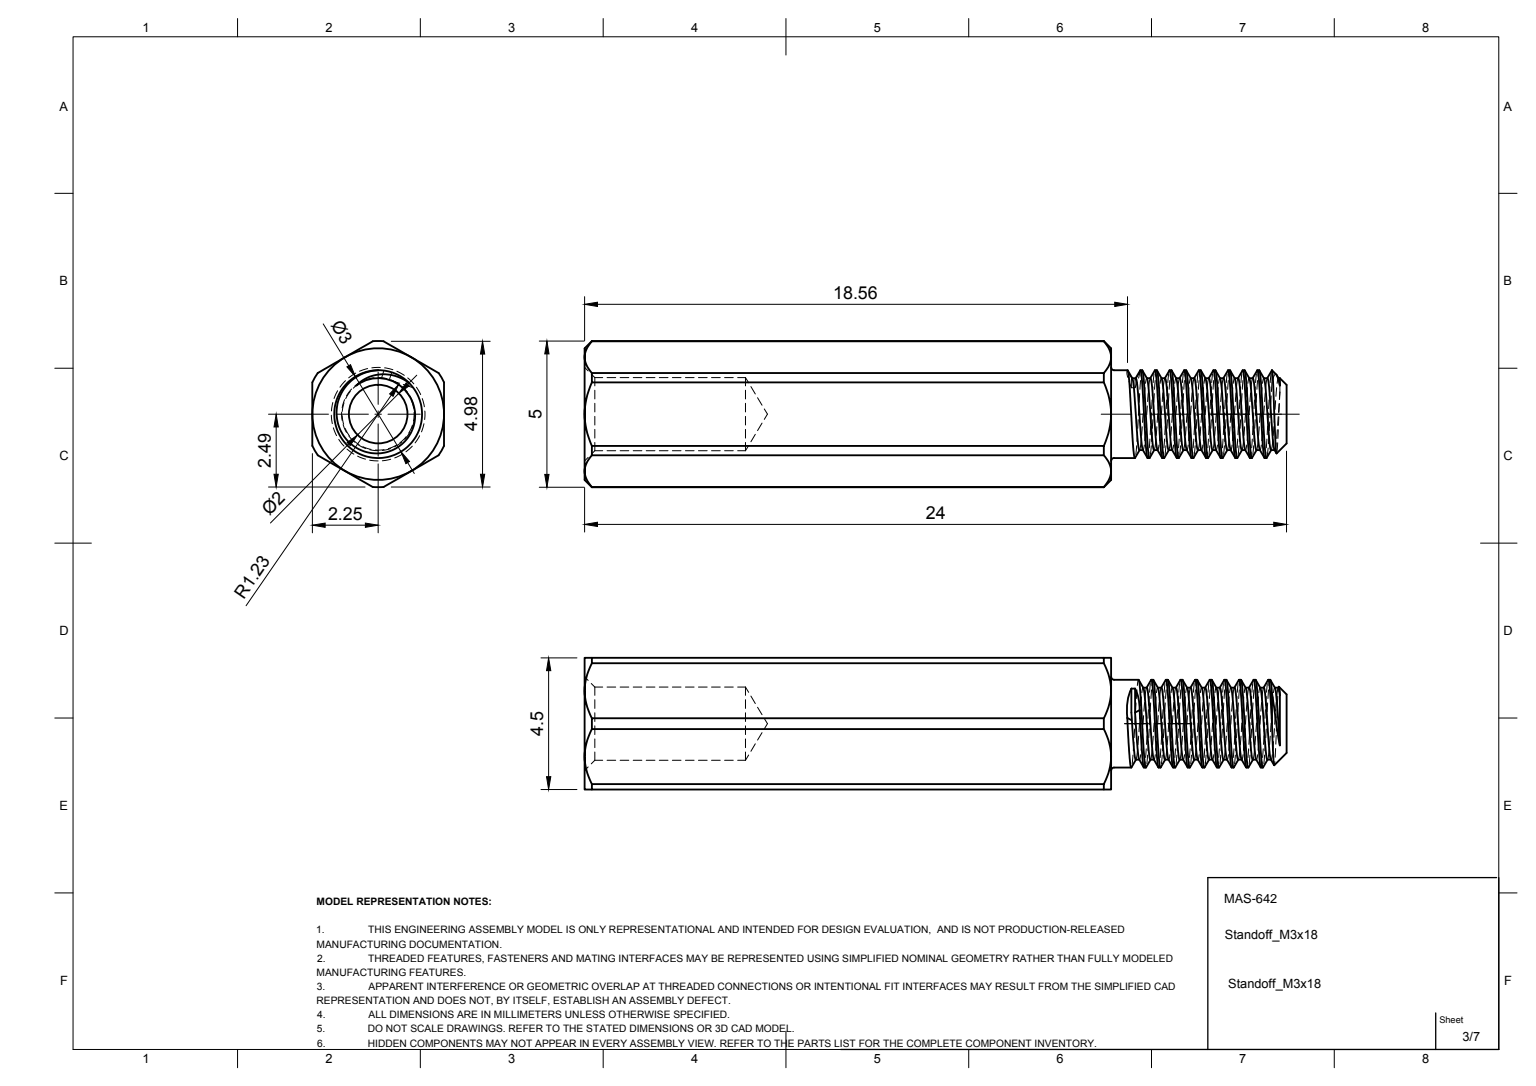
ISO-10303-21;
HEADER;
FILE_DESCRIPTION((''),'2;1');
FILE_NAME('Standoff_M3x18.step','2026-10-09T09:51:33-07:00',(''),(''),'','','');
FILE_SCHEMA (('AUTOMOTIVE_DESIGN { 1 0 10303 214 3 1 1 }'));
ENDSEC;
DATA;
#10=MECHANICAL_DESIGN_GEOMETRIC_PRESENTATION_REPRESENTATION('',(#4170),#126571);
#43=(
BOUNDED_CURVE()
B_SPLINE_CURVE(2,(#125694,#125695,#125696),.UNSPECIFIED.,.F.,.F.)
B_SPLINE_CURVE_WITH_KNOTS((3,3),(2.11928043164924,2.84165444767657),
 .UNSPECIFIED.)
CURVE()
GEOMETRIC_REPRESENTATION_ITEM()
RATIONAL_B_SPLINE_CURVE((4.94937295736919,5.22222222222224,5.22222222222224))
REPRESENTATION_ITEM('')
) ;
#44=(
BOUNDED_CURVE()
B_SPLINE_CURVE(2,(#125699,#125700,#125701),.UNSPECIFIED.,.F.,.F.)
B_SPLINE_CURVE_WITH_KNOTS((3,3),(2.84165444767658,3.56402846370389),
 .UNSPECIFIED.)
CURVE()
GEOMETRIC_REPRESENTATION_ITEM()
RATIONAL_B_SPLINE_CURVE((5.22222222222221,5.22222222222221,4.94937295736917))
REPRESENTATION_ITEM('')
) ;
#45=(
BOUNDED_CURVE()
B_SPLINE_CURVE(2,(#125705,#125706,#125707),.UNSPECIFIED.,.F.,.F.)
B_SPLINE_CURVE_WITH_KNOTS((3,3),(2.84165444767657,3.56402846370389),
 .UNSPECIFIED.)
CURVE()
GEOMETRIC_REPRESENTATION_ITEM()
RATIONAL_B_SPLINE_CURVE((5.22222222222224,5.22222222222224,4.9493729573692))
REPRESENTATION_ITEM('')
) ;
#46=(
BOUNDED_CURVE()
B_SPLINE_CURVE(2,(#125708,#125709,#125710),.UNSPECIFIED.,.F.,.F.)
B_SPLINE_CURVE_WITH_KNOTS((3,3),(2.11928043164924,2.84165444767655),
 .UNSPECIFIED.)
CURVE()
GEOMETRIC_REPRESENTATION_ITEM()
RATIONAL_B_SPLINE_CURVE((4.94937295736915,5.22222222222219,5.22222222222219))
REPRESENTATION_ITEM('')
) ;
#47=(
BOUNDED_CURVE()
B_SPLINE_CURVE(2,(#125714,#125715,#125716),.UNSPECIFIED.,.F.,.F.)
B_SPLINE_CURVE_WITH_KNOTS((3,3),(2.84165444767655,3.56402846370389),
 .UNSPECIFIED.)
CURVE()
GEOMETRIC_REPRESENTATION_ITEM()
RATIONAL_B_SPLINE_CURVE((5.22222222222219,5.22222222222219,4.94937295736914))
REPRESENTATION_ITEM('')
) ;
#48=(
BOUNDED_CURVE()
B_SPLINE_CURVE(2,(#125717,#125718,#125719),.UNSPECIFIED.,.F.,.F.)
B_SPLINE_CURVE_WITH_KNOTS((3,3),(2.11928043164923,2.84165444767657),
 .UNSPECIFIED.)
CURVE()
GEOMETRIC_REPRESENTATION_ITEM()
RATIONAL_B_SPLINE_CURVE((4.94937295736919,5.22222222222224,5.22222222222224))
REPRESENTATION_ITEM('')
) ;
#49=(
BOUNDED_CURVE()
B_SPLINE_CURVE(2,(#125723,#125724,#125725),.UNSPECIFIED.,.F.,.F.)
B_SPLINE_CURVE_WITH_KNOTS((3,3),(2.84165444767657,3.5640284637039),
 .UNSPECIFIED.)
CURVE()
GEOMETRIC_REPRESENTATION_ITEM()
RATIONAL_B_SPLINE_CURVE((5.22222222222224,5.22222222222224,4.94937295736919))
REPRESENTATION_ITEM('')
) ;
#50=(
BOUNDED_CURVE()
B_SPLINE_CURVE(2,(#125726,#125727,#125728),.UNSPECIFIED.,.F.,.F.)
B_SPLINE_CURVE_WITH_KNOTS((3,3),(2.11928043164923,2.84165444767656),
 .UNSPECIFIED.)
CURVE()
GEOMETRIC_REPRESENTATION_ITEM()
RATIONAL_B_SPLINE_CURVE((4.9493729573692,5.22222222222225,5.22222222222225))
REPRESENTATION_ITEM('')
) ;
#51=(
BOUNDED_CURVE()
B_SPLINE_CURVE(2,(#125732,#125733,#125734),.UNSPECIFIED.,.F.,.F.)
B_SPLINE_CURVE_WITH_KNOTS((3,3),(2.84165444767656,3.56402846370389),
 .UNSPECIFIED.)
CURVE()
GEOMETRIC_REPRESENTATION_ITEM()
RATIONAL_B_SPLINE_CURVE((5.22222222222225,5.22222222222225,4.94937295736921))
REPRESENTATION_ITEM('')
) ;
#52=(
BOUNDED_CURVE()
B_SPLINE_CURVE(2,(#125735,#125736,#125737),.UNSPECIFIED.,.F.,.F.)
B_SPLINE_CURVE_WITH_KNOTS((3,3),(2.11928043164924,2.84165444767656),
 .UNSPECIFIED.)
CURVE()
GEOMETRIC_REPRESENTATION_ITEM()
RATIONAL_B_SPLINE_CURVE((4.94937295736916,5.2222222222222,5.2222222222222))
REPRESENTATION_ITEM('')
) ;
#53=(
BOUNDED_CURVE()
B_SPLINE_CURVE(2,(#125740,#125741,#125742),.UNSPECIFIED.,.F.,.F.)
B_SPLINE_CURVE_WITH_KNOTS((3,3),(2.84165444767656,3.56402846370389),
 .UNSPECIFIED.)
CURVE()
GEOMETRIC_REPRESENTATION_ITEM()
RATIONAL_B_SPLINE_CURVE((5.2222222222222,5.2222222222222,4.94937295736915))
REPRESENTATION_ITEM('')
) ;
#54=(
BOUNDED_CURVE()
B_SPLINE_CURVE(2,(#125743,#125744,#125745),.UNSPECIFIED.,.F.,.F.)
B_SPLINE_CURVE_WITH_KNOTS((3,3),(2.11928043164924,2.84165444767658),
 .UNSPECIFIED.)
CURVE()
GEOMETRIC_REPRESENTATION_ITEM()
RATIONAL_B_SPLINE_CURVE((4.94937295736917,5.22222222222221,5.22222222222221))
REPRESENTATION_ITEM('')
) ;
#55=(
BOUNDED_CURVE()
B_SPLINE_CURVE(2,(#125748,#125749,#125750),.UNSPECIFIED.,.F.,.F.)
B_SPLINE_CURVE_WITH_KNOTS((3,3),(2.11928043164923,2.84165444767652),
 .UNSPECIFIED.)
CURVE()
GEOMETRIC_REPRESENTATION_ITEM()
RATIONAL_B_SPLINE_CURVE((4.94937295736913,5.22222222222216,5.22222222222217))
REPRESENTATION_ITEM('')
) ;
#56=(
BOUNDED_CURVE()
B_SPLINE_CURVE(2,(#125753,#125754,#125755),.UNSPECIFIED.,.F.,.F.)
B_SPLINE_CURVE_WITH_KNOTS((3,3),(2.84165444767653,3.56402846370387),
 .UNSPECIFIED.)
CURVE()
GEOMETRIC_REPRESENTATION_ITEM()
RATIONAL_B_SPLINE_CURVE((5.22222222222218,5.22222222222219,4.94937295736914))
REPRESENTATION_ITEM('')
) ;
#57=(
BOUNDED_CURVE()
B_SPLINE_CURVE(2,(#125759,#125760,#125761),.UNSPECIFIED.,.F.,.F.)
B_SPLINE_CURVE_WITH_KNOTS((3,3),(2.84165444767652,3.56402846370389),
 .UNSPECIFIED.)
CURVE()
GEOMETRIC_REPRESENTATION_ITEM()
RATIONAL_B_SPLINE_CURVE((5.22222222222217,5.22222222222218,4.94937295736911))
REPRESENTATION_ITEM('')
) ;
#58=(
BOUNDED_CURVE()
B_SPLINE_CURVE(2,(#125762,#125763,#125764),.UNSPECIFIED.,.F.,.F.)
B_SPLINE_CURVE_WITH_KNOTS((3,3),(2.11928043164923,2.8416544476765),
 .UNSPECIFIED.)
CURVE()
GEOMETRIC_REPRESENTATION_ITEM()
RATIONAL_B_SPLINE_CURVE((4.94937295736913,5.22222222222215,5.22222222222217))
REPRESENTATION_ITEM('')
) ;
#59=(
BOUNDED_CURVE()
B_SPLINE_CURVE(2,(#125766,#125767,#125768),.UNSPECIFIED.,.F.,.F.)
B_SPLINE_CURVE_WITH_KNOTS((3,3),(2.11928043164914,2.84165444767653),
 .UNSPECIFIED.)
CURVE()
GEOMETRIC_REPRESENTATION_ITEM()
RATIONAL_B_SPLINE_CURVE((4.94937295736908,5.22222222222217,5.22222222222218))
REPRESENTATION_ITEM('')
) ;
#60=(
BOUNDED_CURVE()
B_SPLINE_CURVE(2,(#125771,#125772,#125773),.UNSPECIFIED.,.F.,.F.)
B_SPLINE_CURVE_WITH_KNOTS((3,3),(2.84165444767655,3.5640284637039),
 .UNSPECIFIED.)
CURVE()
GEOMETRIC_REPRESENTATION_ITEM()
RATIONAL_B_SPLINE_CURVE((5.22222222222218,5.22222222222218,4.94937295736911))
REPRESENTATION_ITEM('')
) ;
#61=(
BOUNDED_CURVE()
B_SPLINE_CURVE(2,(#125775,#125776,#125777),.UNSPECIFIED.,.F.,.F.)
B_SPLINE_CURVE_WITH_KNOTS((3,3),(2.11928043164924,2.84165444767655),
 .UNSPECIFIED.)
CURVE()
GEOMETRIC_REPRESENTATION_ITEM()
RATIONAL_B_SPLINE_CURVE((4.94937295736915,5.22222222222217,5.22222222222218))
REPRESENTATION_ITEM('')
) ;
#62=(
BOUNDED_CURVE()
B_SPLINE_CURVE(2,(#125780,#125781,#125782),.UNSPECIFIED.,.F.,.F.)
B_SPLINE_CURVE_WITH_KNOTS((3,3),(2.84165444767655,3.56402846370386),
 .UNSPECIFIED.)
CURVE()
GEOMETRIC_REPRESENTATION_ITEM()
RATIONAL_B_SPLINE_CURVE((5.22222222222217,5.22222222222217,4.94937295736913))
REPRESENTATION_ITEM('')
) ;
#63=(
BOUNDED_CURVE()
B_SPLINE_CURVE(2,(#125784,#125785,#125786),.UNSPECIFIED.,.F.,.F.)
B_SPLINE_CURVE_WITH_KNOTS((3,3),(2.11928043164924,2.84165444767655),
 .UNSPECIFIED.)
CURVE()
GEOMETRIC_REPRESENTATION_ITEM()
RATIONAL_B_SPLINE_CURVE((4.94937295736914,5.22222222222217,5.22222222222217))
REPRESENTATION_ITEM('')
) ;
#64=(
BOUNDED_CURVE()
B_SPLINE_CURVE(2,(#125789,#125790,#125791),.UNSPECIFIED.,.F.,.F.)
B_SPLINE_CURVE_WITH_KNOTS((3,3),(2.84165444767657,3.56402846370392),
 .UNSPECIFIED.)
CURVE()
GEOMETRIC_REPRESENTATION_ITEM()
RATIONAL_B_SPLINE_CURVE((5.22222222222219,5.22222222222218,4.94937295736911))
REPRESENTATION_ITEM('')
) ;
#65=(
BOUNDED_CURVE()
B_SPLINE_CURVE(2,(#125793,#125794,#125795),.UNSPECIFIED.,.F.,.F.)
B_SPLINE_CURVE_WITH_KNOTS((3,3),(2.11928043164923,2.84165444767657),
 .UNSPECIFIED.)
CURVE()
GEOMETRIC_REPRESENTATION_ITEM()
RATIONAL_B_SPLINE_CURVE((4.94937295736915,5.2222222222222,5.22222222222219))
REPRESENTATION_ITEM('')
) ;
#66=(
BOUNDED_CURVE()
B_SPLINE_CURVE(2,(#125797,#125798,#125799),.UNSPECIFIED.,.F.,.F.)
B_SPLINE_CURVE_WITH_KNOTS((3,3),(2.8416544476765,3.56402846370386),
 .UNSPECIFIED.)
CURVE()
GEOMETRIC_REPRESENTATION_ITEM()
RATIONAL_B_SPLINE_CURVE((5.22222222222217,5.22222222222219,4.94937295736913))
REPRESENTATION_ITEM('')
) ;
#330=B_SPLINE_CURVE_WITH_KNOTS('',3,(#124047,#124048,#124049,#124050,#124051,
#124052,#124053,#124054,#124055,#124056,#124057,#124058,#124059,#124060,
#124061,#124062,#124063,#124064,#124065,#124066),.UNSPECIFIED.,.F.,.F.,
(4,2,2,2,2,2,2,2,2,4),(7.26097235916453,7.307487976323,7.35575594389105,
7.40257156416353,7.45158020939779,7.49931815600202,7.54681878982848,7.59584329786992,
7.64302175237609,7.68775617947263),.UNSPECIFIED.) ;
#331=B_SPLINE_CURVE_WITH_KNOTS('',3,(#124069,#124070,#124071,#124072,#124073,
#124074,#124075,#124076,#124077,#124078,#124079,#124080,#124081,#124082,
#124083,#124084,#124085,#124086,#124087,#124088),.UNSPECIFIED.,.F.,.F.,
(4,2,2,2,2,2,2,2,2,4),(0.,0.0459875521653835,0.0932819628997698,0.142429322852028,
0.189908590414643,0.237761664358612,0.28683868989661,0.333704279409584,
0.382086034209551,0.427411498485805),.UNSPECIFIED.) ;
#332=B_SPLINE_CURVE_WITH_KNOTS('',3,(#124093,#124094,#124095,#124096,#124097,
#124098,#124099,#124100,#124101,#124102,#124103,#124104,#124105,#124106,
#124107,#124108,#124109,#124110,#124111,#124112,#124113,#124114,#124115,
#124116,#124117,#124118,#124119,#124120,#124121,#124122,#124123,#124124,
#124125,#124126,#124127,#124128,#124129,#124130),.UNSPECIFIED.,.F.,.F.,
(4,2,2,2,2,2,2,2,2,2,2,2,2,2,2,2,2,2,4),(6.48467832939662,6.48870478558093,
6.53766507492409,6.58568550492772,6.63267823725172,6.68202082324882,6.72948815834683,
6.77759017644729,6.82630561099994,6.87323621682889,6.92225205593385,6.97046423370673,
7.01740641521615,7.06695661317869,7.11461532958629,7.16247212938834,7.21140015580506,
7.25849183169839,7.26097235916453),.UNSPECIFIED.) ;
#333=B_SPLINE_CURVE_WITH_KNOTS('',3,(#124131,#124132,#124133,#124134,#124135,
#124136,#124137,#124138,#124139,#124140,#124141,#124142,#124143,#124144,
#124145,#124146,#124147,#124148,#124149,#124150,#124151,#124152,#124153,
#124154,#124155,#124156,#124157,#124158,#124159,#124160,#124161,#124162,
#124163,#124164,#124165,#124166,#124167,#124168),.UNSPECIFIED.,.F.,.F.,
(4,2,2,2,2,2,2,2,2,2,2,2,2,2,2,2,2,2,4),(0.427411498485805,0.431577036060463,
0.478789185503758,0.527845315274495,0.575603226460443,0.623379302822146,
0.672502619127436,0.719463017877226,0.767773403599721,0.816880465796082,
0.864021613138868,0.912997981216,0.961170824102338,1.00888581090197,1.0584891685082,
1.10562630736056,1.1538964673421,1.20305610785317,1.20577246230604),
 .UNSPECIFIED.) ;
#334=B_SPLINE_CURVE_WITH_KNOTS('',3,(#124173,#124174,#124175,#124176,#124177,
#124178,#124179,#124180,#124181,#124182,#124183,#124184,#124185,#124186,
#124187,#124188,#124189,#124190,#124191,#124192,#124193,#124194,#124195,
#124196,#124197,#124198,#124199,#124200,#124201,#124202,#124203,#124204,
#124205,#124206,#124207,#124208),.UNSPECIFIED.,.F.,.F.,(4,2,2,2,2,2,2,2,
2,2,2,2,2,2,2,2,2,4),(5.70956420747771,5.72030972034507,5.76926273175053,
5.81700561122586,5.86434645191125,5.91338162506858,5.96056756496257,6.00942404361783,
6.05780748008125,6.10453345170252,6.15347366016584,6.20133669000566,6.24846500640859,
6.29763501900576,6.34494399136913,6.39338455386973,6.4419176261338,6.48467832939662),
 .UNSPECIFIED.) ;
#335=B_SPLINE_CURVE_WITH_KNOTS('',3,(#124209,#124210,#124211,#124212,#124213,
#124214,#124215,#124216,#124217,#124218,#124219,#124220,#124221,#124222,
#124223,#124224,#124225,#124226,#124227,#124228,#124229,#124230,#124231,
#124232,#124233,#124234,#124235,#124236,#124237,#124238,#124239,#124240,
#124241,#124242,#124243,#124244),.UNSPECIFIED.,.F.,.F.,(4,2,2,2,2,2,2,2,
2,2,2,2,2,2,2,2,2,4),(1.20577246230604,1.2500637087132,1.29884493426391,
1.34732241102889,1.39486523697925,1.44428132500633,1.49152186175626,1.53962022531109,
1.58874613172205,1.63565991568587,1.68427775017929,1.73314474249065,1.78054992698739,
1.8298155429656,1.87724047764212,1.92520328493819,1.97432941645622,1.98383043851811),
 .UNSPECIFIED.) ;
#336=B_SPLINE_CURVE_WITH_KNOTS('',3,(#124249,#124250,#124251,#124252,#124253,
#124254,#124255,#124256,#124257,#124258,#124259,#124260,#124261,#124262,
#124263,#124264,#124265,#124266,#124267,#124268,#124269,#124270,#124271,
#124272,#124273,#124274,#124275,#124276,#124277,#124278,#124279,#124280,
#124281,#124282,#124283,#124284),.UNSPECIFIED.,.F.,.F.,(4,2,2,2,2,2,2,2,
2,2,2,2,2,2,2,2,2,4),(4.93350849726113,4.95065313897434,5.0001367514161,
5.04773589353637,5.09575665066723,5.14461540943155,5.19164298059034,5.24062387411831,
5.28881904095715,5.33565288934101,5.38464956624476,5.43231220009687,5.4799267516029,
5.52886743736441,5.57596806240929,5.62529535397539,5.67356510724699,5.70956420747771),
 .UNSPECIFIED.) ;
#337=B_SPLINE_CURVE_WITH_KNOTS('',3,(#124285,#124286,#124287,#124288,#124289,
#124290,#124291,#124292,#124293,#124294,#124295,#124296,#124297,#124298,
#124299,#124300,#124301,#124302,#124303,#124304,#124305,#124306,#124307,
#124308,#124309,#124310,#124311,#124312,#124313,#124314,#124315,#124316,
#124317,#124318,#124319,#124320),.UNSPECIFIED.,.F.,.F.,(4,2,2,2,2,2,2,2,
2,2,2,2,2,2,2,2,2,4),(1.98383043851811,2.021231364205,2.0697205926988,2.11904155289011,
2.1663460448574,2.21550071170308,2.26317878691631,2.31104512794968,2.36020318829153,
2.40716845964159,2.4555671563287,2.50471172270157,2.55193271124501,2.60099435417148,
2.64904317691366,2.69683410923425,2.74652048876617,2.76242745970405),
 .UNSPECIFIED.) ;
#338=B_SPLINE_CURVE_WITH_KNOTS('',3,(#124325,#124326,#124327,#124328,#124329,
#124330,#124331,#124332,#124333,#124334,#124335,#124336,#124337,#124338,
#124339,#124340,#124341,#124342,#124343,#124344,#124345,#124346,#124347,
#124348,#124349,#124350,#124351,#124352,#124353,#124354,#124355,#124356,
#124357,#124358,#124359,#124360),.UNSPECIFIED.,.F.,.F.,(4,2,2,2,2,2,2,2,
2,2,2,2,2,2,2,2,2,4),(4.15738429453256,4.18139819511275,4.23053919796976,
4.27782394869024,4.32652355399284,4.37501975350424,4.42180928210789,4.47080187820887,
4.51878063593279,4.56588041443636,4.61517448159553,4.66259930855119,4.71091650689067,
4.7595782551651,4.80646789213435,4.8554969233847,4.90364974207811,4.93350849726113),
 .UNSPECIFIED.) ;
#339=B_SPLINE_CURVE_WITH_KNOTS('',3,(#124361,#124362,#124363,#124364,#124365,
#124366,#124367,#124368,#124369,#124370,#124371,#124372,#124373,#124374,
#124375,#124376,#124377,#124378,#124379,#124380,#124381,#124382,#124383,
#124384,#124385,#124386,#124387,#124388,#124389,#124390,#124391,#124392,
#124393,#124394,#124395,#124396),.UNSPECIFIED.,.F.,.F.,(4,2,2,2,2,2,2,2,
2,2,2,2,2,2,2,2,2,4),(2.76242745970405,2.7936241020587,2.84197026691353,
2.89114229506907,2.93820657938614,2.98705917484022,3.03536824467617,3.08297180498013,
3.13245479128841,3.17962172814637,3.22778030392872,3.27690191435427,3.32383405210944,
3.3725082345208,3.421169403163,3.46861903657913,3.51793416507266,3.54067593133588),
 .UNSPECIFIED.) ;
#340=B_SPLINE_CURVE_WITH_KNOTS('',3,(#124401,#124402,#124403,#124404,#124405,
#124406,#124407,#124408,#124409,#124410,#124411,#124412,#124413,#124414,
#124415,#124416,#124417,#124418,#124419,#124420,#124421,#124422,#124423,
#124424,#124425,#124426,#124427,#124428,#124429,#124430,#124431,#124432,
#124433,#124434,#124435,#124436),.UNSPECIFIED.,.F.,.F.,(4,2,2,2,2,2,2,2,
2,2,2,2,2,2,2,2,2,4),(3.3811260484289,3.41274900862816,3.46099351805033,
3.51004032645083,3.55700214539487,3.60575007739184,3.65387741150041,3.70137616908567,
3.75075153504194,3.79777167498976,3.84582386285438,3.89300519478398,3.94215330243098,
3.99051838064245,4.03728979359576,4.08628002368325,4.13412062890419,4.15738429453256),
 .UNSPECIFIED.) ;
#341=B_SPLINE_CURVE_WITH_KNOTS('',3,(#124437,#124438,#124439,#124440,#124441,
#124442,#124443,#124444,#124445,#124446,#124447,#124448,#124449,#124450,
#124451,#124452,#124453,#124454,#124455,#124456,#124457,#124458,#124459,
#124460,#124461,#124462,#124463,#124464,#124465,#124466,#124467,#124468,
#124469,#124470,#124471,#124472),.UNSPECIFIED.,.F.,.F.,(4,2,2,2,2,2,2,2,
2,2,2,2,2,2,2,2,2,4),(3.54067593133588,3.56524889916681,3.6132547608121,
3.66236113995851,3.70924379097633,3.75777283633892,3.80686079772826,3.85419230870826,
3.90337783950468,3.95091591719774,4.0002920934568,4.0477975955105,4.09630989433075,
4.14504988690739,4.19202367440407,4.2411602470478,4.2893880427099,4.31858521036147),
 .UNSPECIFIED.) ;
#342=B_SPLINE_CURVE_WITH_KNOTS('',3,(#124477,#124478,#124479,#124480,#124481,
#124482,#124483,#124484,#124485,#124486,#124487,#124488,#124489,#124490,
#124491,#124492,#124493,#124494,#124495,#124496,#124497,#124498,#124499,
#124500,#124501,#124502,#124503,#124504,#124505,#124506,#124507,#124508,
#124509,#124510,#124511,#124512),.UNSPECIFIED.,.F.,.F.,(4,2,2,2,2,2,2,2,
2,2,2,2,2,2,2,2,2,4),(2.60440000418254,2.64222091806599,2.69061789859203,
2.73975515555105,2.78696572159386,2.83602367520873,2.88355189021403,2.93132224967008,
2.98036249985887,3.02720769453067,3.07550834816351,3.12453618250826,3.17165958350625,
3.22062064308854,3.26850397351192,3.31619467232154,3.36577824481598,3.3811260484289),
 .UNSPECIFIED.) ;
#343=B_SPLINE_CURVE_WITH_KNOTS('',3,(#124513,#124514,#124515,#124516,#124517,
#124518,#124519,#124520,#124521,#124522,#124523,#124524,#124525,#124526,
#124527,#124528,#124529,#124530,#124531,#124532,#124533,#124534,#124535,
#124536,#124537,#124538,#124539,#124540,#124541,#124542,#124543,#124544,
#124545,#124546,#124547,#124548),.UNSPECIFIED.,.F.,.F.,(4,2,2,2,2,2,2,2,
2,2,2,2,2,2,2,2,2,4),(4.31858521036147,4.33651923363743,4.38607754453018,
4.43375037804094,4.48194507407388,4.53087577616931,4.57797363563567,4.62704987194849,
4.67531370070556,4.72225592255632,4.77134912087816,4.81907824427662,4.86684436513085,
4.91585036470624,4.96301502121423,5.01254217112715,5.06087102345235,5.09618003538743),
 .UNSPECIFIED.) ;
#344=B_SPLINE_CURVE_WITH_KNOTS('',3,(#124553,#124554,#124555,#124556,#124557,
#124558,#124559,#124560,#124561,#124562,#124563,#124564,#124565,#124566,
#124567,#124568,#124569,#124570,#124571,#124572,#124573,#124574,#124575,
#124576,#124577,#124578,#124579,#124580,#124581,#124582,#124583,#124584,
#124585,#124586,#124587,#124588),.UNSPECIFIED.,.F.,.F.,(4,2,2,2,2,2,2,2,
2,2,2,2,2,2,2,2,2,4),(1.82805130471776,1.87277646127533,1.92147530871624,
1.96979104419725,2.01725060263876,2.06658135847983,2.11369404932703,2.16170773952795,
2.2107256291696,2.25754243281317,2.30607324540708,2.35476584472025,2.40208265835429,
2.45125749765287,2.49854231366641,2.54641504154563,2.59542814286478,2.60440000418254),
 .UNSPECIFIED.) ;
#345=B_SPLINE_CURVE_WITH_KNOTS('',3,(#124589,#124590,#124591,#124592,#124593,
#124594,#124595,#124596,#124597,#124598,#124599,#124600,#124601,#124602,
#124603,#124604,#124605,#124606,#124607,#124608,#124609,#124610,#124611,
#124612,#124613,#124614,#124615,#124616,#124617,#124618,#124619,#124620,
#124621,#124622,#124623,#124624),.UNSPECIFIED.,.F.,.F.,(4,2,2,2,2,2,2,2,
2,2,2,2,2,2,2,2,2,4),(5.09618003538743,5.10770893818563,5.15675128793345,
5.20455098500115,5.25203122076791,5.3011219283047,5.34836274788015,5.39740888690433,
5.44584255805835,5.49264392480102,5.54166593188317,5.58957668485638,5.63682763234505,
5.68604400914993,5.73339928464143,5.78201352428103,5.8305888160979,5.8725887638988),
 .UNSPECIFIED.) ;
#346=B_SPLINE_CURVE_WITH_KNOTS('',3,(#124629,#124630,#124631,#124632,#124633,
#124634,#124635,#124636,#124637,#124638,#124639,#124640,#124641,#124642,
#124643,#124644,#124645,#124646,#124647,#124648,#124649,#124650,#124651,
#124652,#124653,#124654,#124655,#124656,#124657,#124658,#124659,#124660,
#124661,#124662,#124663,#124664,#124665,#124666),.UNSPECIFIED.,.F.,.F.,
(4,2,2,2,2,2,2,2,2,2,2,2,2,2,2,2,2,2,4),(1.05122908753305,1.05584848690386,
1.10298878125772,1.15197109295181,1.19959776737697,1.24730001658321,1.29632817220458,
1.34318726064785,1.39142201535752,1.44043479373918,1.48749995499297,1.536398131184,
1.58442418882633,1.63206057663025,1.68158354821496,1.72860610089148,1.77679646385941,
1.82585341919623,1.82805130471776),.UNSPECIFIED.) ;
#347=B_SPLINE_CURVE_WITH_KNOTS('',3,(#124667,#124668,#124669,#124670,#124671,
#124672,#124673,#124674,#124675,#124676,#124677,#124678,#124679,#124680,
#124681,#124682,#124683,#124684,#124685,#124686,#124687,#124688,#124689,
#124690,#124691,#124692,#124693,#124694,#124695,#124696,#124697,#124698,
#124699,#124700,#124701,#124702,#124703,#124704),.UNSPECIFIED.,.F.,.F.,
(4,2,2,2,2,2,2,2,2,2,2,2,2,2,2,2,2,2,4),(5.8725887638988,5.87743194290884,
5.92646601185683,5.97452581587684,6.02162175582692,6.07100225132472,6.11850795426233,
6.1667628942196,6.21551331591218,6.2624807124907,6.31156171305631,6.35980565105167,
6.40683027516766,6.456410610302,6.50410033527444,6.55208641404564,6.6010427526743,
6.64816284268059,6.64991209706395),.UNSPECIFIED.) ;
#348=B_SPLINE_CURVE_WITH_KNOTS('',3,(#124709,#124710,#124711,#124712,#124713,
#124714,#124715,#124716,#124717,#124718,#124719,#124720,#124721,#124722,
#124723,#124724,#124725,#124726,#124727,#124728,#124729,#124730,#124731,
#124732,#124733,#124734,#124735,#124736,#124737,#124738,#124739,#124740,
#124741,#124742,#124743,#124744),.UNSPECIFIED.,.F.,.F.,(4,2,2,2,2,2,2,2,
2,2,2,2,2,2,2,2,2,4),(0.275540243682509,0.286340819800539,0.333695388575774,
0.382913371187234,0.430062940631542,0.477971836820167,0.526948240257121,
0.573710230464671,0.622139368966846,0.670997426602599,0.718226071803216,
0.767306120243138,0.814662887431798,0.862448581964833,0.911435350682647,
0.958210116723726,1.00652260961773,1.05122908753305),.UNSPECIFIED.) ;
#349=B_SPLINE_CURVE_WITH_KNOTS('',3,(#124745,#124746,#124747,#124748,#124749,
#124750,#124751,#124752,#124753,#124754,#124755,#124756,#124757,#124758,
#124759,#124760,#124761,#124762,#124763,#124764,#124765,#124766,#124767,
#124768,#124769,#124770,#124771,#124772,#124773,#124774,#124775,#124776,
#124777,#124778,#124779,#124780),.UNSPECIFIED.,.F.,.F.,(4,2,2,2,2,2,2,2,
2,2,2,2,2,2,2,2,2,4),(6.64991209706395,6.69721143233729,6.74550549456067,
6.79238454552838,6.84144720027061,6.88920947529323,6.93681673187035,6.98586340790173,
7.03306447569406,7.08232935533034,7.13071011437757,7.17751961704142,7.22654758629657,
7.27440241377778,7.32175171314648,7.37090535322958,7.41820339493711,7.42653426035933),
 .UNSPECIFIED.) ;
#350=B_SPLINE_CURVE_WITH_KNOTS('',3,(#124786,#124787,#124788,#124789,#124790,
#124791,#124792,#124793,#124794,#124795,#124796,#124797),.UNSPECIFIED.,
 .F.,.F.,(4,2,2,2,2,4),(-0.236473027122006,-0.23458695710018,-0.176673006834002,
-0.118290109209632,-0.0588288584469845,-1.00000016489687E-6),
 .UNSPECIFIED.) ;
#351=B_SPLINE_CURVE_WITH_KNOTS('',3,(#124800,#124801,#124802,#124803,#124804,
#124805,#124806,#124807),.UNSPECIFIED.,.F.,.F.,(4,2,2,4),(-9.35462171155631,
-9.30382148989728,-9.24635104762449,-9.23530418985942),.UNSPECIFIED.) ;
#352=B_SPLINE_CURVE_WITH_KNOTS('',3,(#124812,#124813,#124814,#124815,#124816,
#124817,#124818,#124819,#124820,#124821,#124822,#124823,#124824,#124825,
#124826,#124827,#124828,#124829,#124830,#124831,#124832,#124833,#124834,
#124835,#124836,#124837,#124838,#124839,#124840,#124841,#124842,#124843,
#124844,#124845,#124846,#124847),.UNSPECIFIED.,.F.,.F.,(4,2,2,2,2,2,2,2,
2,2,2,2,2,2,2,2,2,4),(-1.1816466799126,-1.1711432489464,-1.11360549897867,
-1.05429971803153,-0.99527231100603,-0.938324784610826,-0.878701151729204,
-0.820319907036438,-0.763004488472792,-0.70301164166561,-0.645300597460547,
-0.586507743434059,-0.527276575096228,-0.470213578625258,-0.410561930645358,
-0.351974482019793,-0.294804872599786,-0.236473027122006),.UNSPECIFIED.) ;
#353=B_SPLINE_CURVE_WITH_KNOTS('',3,(#124848,#124849,#124850,#124851,#124852,
#124853,#124854,#124855,#124856,#124857,#124858,#124859,#124860,#124861,
#124862,#124863,#124864,#124865,#124866,#124867,#124868,#124869,#124870,
#124871,#124872,#124873,#124874,#124875,#124876,#124877,#124878,#124879,
#124880,#124881,#124882,#124883),.UNSPECIFIED.,.F.,.F.,(4,2,2,2,2,2,2,2,
2,2,2,2,2,2,2,2,2,4),(-9.23530418985942,-9.18662207546147,-9.1290733058091,
-9.07093314408142,-9.01135436272492,-8.95446571047789,-8.89567746304653,
-8.83575191467067,-8.77841492190154,-8.71883583043751,-8.66095591767163,
-8.60294688747092,-8.54333582365895,-8.48636391838879,-8.42770437782455,
-8.3681122074522,-8.31090295919035,-8.29087925177368),.UNSPECIFIED.) ;
#354=B_SPLINE_CURVE_WITH_KNOTS('',3,(#124888,#124889,#124890,#124891,#124892,
#124893,#124894,#124895,#124896,#124897,#124898,#124899,#124900,#124901,
#124902,#124903,#124904,#124905,#124906,#124907,#124908,#124909,#124910,
#124911,#124912,#124913,#124914,#124915,#124916,#124917,#124918,#124919,
#124920,#124921,#124922,#124923),.UNSPECIFIED.,.F.,.F.,(4,2,2,2,2,2,2,2,
2,2,2,2,2,2,2,2,2,4),(-2.12678122509193,-2.10729425304151,-2.05002580839115,
-1.99038909831469,-1.9316674048963,-1.87466417496185,-1.81501013841361,
-1.75693914324514,-1.69905824232611,-1.63941349055435,-1.58201455193184,
-1.52211994070396,-1.46326421662004,-1.40633380819462,-1.34670866487524,
-1.28850127053106,-1.2309432907053,-1.1816466799126),.UNSPECIFIED.) ;
#355=B_SPLINE_CURVE_WITH_KNOTS('',3,(#124924,#124925,#124926,#124927,#124928,
#124929,#124930,#124931,#124932,#124933,#124934,#124935,#124936,#124937,
#124938,#124939,#124940,#124941,#124942,#124943,#124944,#124945,#124946,
#124947,#124948,#124949,#124950,#124951,#124952,#124953,#124954,#124955,
#124956,#124957,#124958,#124959),.UNSPECIFIED.,.F.,.F.,(4,2,2,2,2,2,2,2,
2,2,2,2,2,2,2,2,2,4),(-8.29087925177368,-8.25146774569309,-8.1931060140114,
-8.1352172805656,-8.07502593792519,-8.01787916182783,-7.95931748219078,
-7.89969072165382,-7.84265244666734,-7.78344729198975,-7.72467517694015,
-7.66698930483589,-7.60702272505567,-7.5497294421654,-7.4913736598247,-7.43177467302502,
-7.37485108389259,-7.3459015110284),.UNSPECIFIED.) ;
#356=B_SPLINE_CURVE_WITH_KNOTS('',3,(#124964,#124965,#124966,#124967,#124968,
#124969,#124970,#124971,#124972,#124973,#124974,#124975,#124976,#124977,
#124978,#124979,#124980,#124981,#124982,#124983,#124984,#124985,#124986,
#124987,#124988,#124989,#124990,#124991,#124992,#124993,#124994,#124995,
#124996,#124997,#124998,#124999),.UNSPECIFIED.,.F.,.F.,(4,2,2,2,2,2,2,2,
2,2,2,2,2,2,2,2,2,4),(-3.07234930182782,-3.04396460692137,-2.98700170532857,
-2.92736930082992,-2.86895787619047,-2.81165872476739,-2.7516332217495,
-2.69389232736989,-2.63514802811358,-2.5758833604033,-2.51879305661577,
-2.45912888472762,-2.40050767619665,-2.34334201878956,-2.28308786627346,
-2.22514048990784,-2.16679217042194,-2.12678122509193),.UNSPECIFIED.) ;
#357=B_SPLINE_CURVE_WITH_KNOTS('',3,(#125000,#125001,#125002,#125003,#125004,
#125005,#125006,#125007,#125008,#125009,#125010,#125011,#125012,#125013,
#125014,#125015,#125016,#125017,#125018,#125019,#125020,#125021,#125022,
#125023,#125024,#125025,#125026,#125027,#125028,#125029,#125030,#125031,
#125032,#125033,#125034,#125035),.UNSPECIFIED.,.F.,.F.,(4,2,2,2,2,2,2,2,
2,2,2,2,2,2,2,2,2,4),(-7.3459015110284,-7.31584938880444,-7.25656387817681,
-7.19905098889278,-7.13927687406326,-7.08174045168678,-7.02355818700801,
-6.9639574791867,-6.90705028583207,-6.84821994204823,-6.78834540215938,
-6.73097099328063,-6.67135180647426,-6.61349209399495,-6.55544587606107,
-6.49581608898128,-6.43883548963137,-6.40128325260829),.UNSPECIFIED.) ;
#358=B_SPLINE_CURVE_WITH_KNOTS('',3,(#125040,#125041,#125042,#125043,#125044,
#125045,#125046,#125047,#125048,#125049,#125050,#125051,#125052,#125053,
#125054,#125055,#125056,#125057,#125058,#125059,#125060,#125061,#125062,
#125063,#125064,#125065,#125066,#125067,#125068,#125069,#125070,#125071,
#125072,#125073,#125074,#125075),.UNSPECIFIED.,.F.,.F.,(4,2,2,2,2,2,2,2,
2,2,2,2,2,2,2,2,2,4),(-4.01743446108088,-3.98037711695305,-3.92338026613865,
-3.86372411788194,-3.80563194583232,-3.74778671319995,-3.68811833045966,
-3.63069784236149,-3.57087032386455,-3.51198882129594,-3.45505470154523,
-3.39542422850156,-3.33719086850357,-3.27966026017497,-3.21983177136984,
-3.1622680481908,-3.10302199988204,-3.07234930182782),.UNSPECIFIED.) ;
#359=B_SPLINE_CURVE_WITH_KNOTS('',3,(#125076,#125077,#125078,#125079,#125080,
#125081,#125082,#125083,#125084,#125085,#125086,#125087,#125088,#125089,
#125090,#125091,#125092,#125093,#125094,#125095,#125096,#125097,#125098,
#125099,#125100,#125101,#125102,#125103,#125104,#125105,#125106,#125107,
#125108,#125109,#125110,#125111),.UNSPECIFIED.,.F.,.F.,(4,2,2,2,2,2,2,2,
2,2,2,2,2,2,2,2,2,4),(-6.40128325260829,-6.38013882187402,-6.32052644786668,
-6.26328232847502,-6.20380975384858,-6.14548195466263,-6.08755912059145,
-6.0273305946859,-5.97018690671393,-5.91159053837258,-5.85195029651196,
-5.79488386817085,-5.73564427374236,-5.67691979083501,-5.61920315388539,
-5.5592029693765,-5.50192507313698,-5.45600166496054),.UNSPECIFIED.) ;
#360=B_SPLINE_CURVE_WITH_KNOTS('',3,(#125116,#125117,#125118,#125119,#125120,
#125121,#125122,#125123,#125124,#125125,#125126,#125127,#125128,#125129,
#125130,#125131,#125132,#125133,#125134,#125135,#125136,#125137,#125138,
#125139,#125140,#125141,#125142,#125143,#125144,#125145,#125146,#125147,
#125148,#125149,#125150,#125151),.UNSPECIFIED.,.F.,.F.,(4,2,2,2,2,2,2,2,
2,2,2,2,2,2,2,2,2,4),(-4.96307563769018,-4.91813866664957,-4.86025738965345,
-4.80218793930441,-4.74253483237101,-4.68553219539954,-4.62681204815797,
-4.5671763186103,-4.50990933760739,-4.45041297938131,-4.3920638222817,-4.33411788796424,
-4.27386529354949,-4.21556664620729,-4.15604769936401,-4.0987601299753,
-4.03911975185839,-4.01743446108088),.UNSPECIFIED.) ;
#361=B_SPLINE_CURVE_WITH_KNOTS('',3,(#125152,#125153,#125154,#125155,#125156,
#125157,#125158,#125159,#125160,#125161,#125162,#125163,#125164,#125165,
#125166,#125167,#125168,#125169,#125170,#125171,#125172,#125173,#125174,
#125175,#125176,#125177,#125178,#125179,#125180,#125181,#125182,#125183,
#125184,#125185,#125186,#125187),.UNSPECIFIED.,.F.,.F.,(4,2,2,2,2,2,2,2,
2,2,2,2,2,2,2,2,2,4),(-5.45600166496054,-5.44353818748178,-5.38392946676581,
-5.32698965292687,-5.26795703729325,-5.20873029520478,-5.15119052229069,
-5.09138701680441,-5.03387705745448,-4.97566790823344,-4.916060903816,-4.85914913392717,
-4.80029208196713,-4.74048362398375,-4.68308675803797,-4.62463408755934,
-4.56743411515897,-4.51134022964834),.UNSPECIFIED.) ;
#362=B_SPLINE_CURVE_WITH_KNOTS('',3,(#125192,#125193,#125194,#125195,#125196,
#125197,#125198,#125199,#125200,#125201,#125202,#125203,#125204,#125205,
#125206,#125207,#125208,#125209,#125210,#125211,#125212,#125213,#125214,
#125215,#125216,#125217,#125218,#125219,#125220,#125221,#125222,#125223,
#125224,#125225,#125226,#125227),.UNSPECIFIED.,.F.,.F.,(4,2,2,2,2,2,2,2,
2,2,2,2,2,2,2,2,2,4),(-5.90797790587752,-5.85417655914304,-5.79686139893281,
-5.73848200916043,-5.67885952882914,-5.62191332079682,-5.56288777161221,
-5.50358081908249,-5.44604476955684,-5.38624654359381,-5.32868845608922,
-5.27048277087713,-5.21085866475879,-5.15392918370283,-5.0950751718008,
-5.03517915849782,-4.97778176824204,-4.96307563769018),.UNSPECIFIED.) ;
#363=B_SPLINE_CURVE_WITH_KNOTS('',3,(#125228,#125229,#125230,#125231,#125232,
#125233,#125234,#125235,#125236,#125237,#125238,#125239,#125240,#125241,
#125242,#125243,#125244,#125245,#125246,#125247,#125248,#125249,#125250,
#125251,#125252,#125253,#125254,#125255,#125256,#125257,#125258,#125259,
#125260,#125261,#125262,#125263,#125264,#125265),.UNSPECIFIED.,.F.,.F.,
(4,2,2,2,2,2,2,2,2,2,2,2,2,2,2,2,2,2,4),(-4.51134022964834,-4.50736107889285,
-4.44957955522536,-4.39103805795909,-4.33172296596087,-4.27459313534948,
-4.21494515138725,-4.15627197557177,-4.09916570838644,-4.03885333731966,
-3.98085531235153,-3.92266438621144,-3.86310737388169,-3.80578556710095,
-3.74614371498309,-3.68736332860037,-3.63038329021729,-3.57072909156752,
-3.56587391815655),.UNSPECIFIED.) ;
#364=B_SPLINE_CURVE_WITH_KNOTS('',3,(#125270,#125271,#125272,#125273,#125274,
#125275,#125276,#125277,#125278,#125279,#125280,#125281,#125282,#125283,
#125284,#125285,#125286,#125287,#125288,#125289,#125290,#125291,#125292,
#125293,#125294,#125295,#125296,#125297,#125298,#125299,#125300,#125301,
#125302,#125303,#125304,#125305,#125306,#125307),.UNSPECIFIED.,.F.,.F.,
(4,2,2,2,2,2,2,2,2,2,2,2,2,2,2,2,2,2,4),(-6.85333016178901,-6.85049761572826,
-6.79086280145887,-6.7338684673792,-6.67518502916102,-6.61556907483254,
-6.55833655807044,-6.49887713904935,-6.44049363778125,-6.38258139356379,
-6.32236555670732,-6.26519661684873,-6.20661114802352,-6.14696077866283,
-6.08989950504226,-6.03067031724312,-5.97187665370647,-5.91416744423235,
-5.90797790587752),.UNSPECIFIED.) ;
#365=B_SPLINE_CURVE_WITH_KNOTS('',3,(#125308,#125309,#125310,#125311,#125312,
#125313,#125314,#125315,#125316,#125317,#125318,#125319,#125320,#125321,
#125322,#125323,#125324,#125325,#125326,#125327,#125328,#125329,#125330,
#125331,#125332,#125333,#125334,#125335,#125336,#125337,#125338,#125339,
#125340,#125341,#125342,#125343),.UNSPECIFIED.,.F.,.F.,(4,2,2,2,2,2,2,2,
2,2,2,2,2,2,2,2,2,4),(-3.56587391815655,-3.51259862586625,-3.4548315841227,
-3.39512002261551,-3.33766052431138,-3.27797683666954,-3.21904783493571,
-3.16210893490559,-3.10247369370918,-3.04419237234846,-2.98672132744669,
-2.92683995638948,-2.86922830950958,-2.8101092431121,-2.75099595568126,
-2.69400388512544,-2.63435950322405,-2.62073726926079),.UNSPECIFIED.) ;
#366=B_SPLINE_CURVE_WITH_KNOTS('',3,(#125350,#125351,#125352,#125353,#125354,
#125355,#125356,#125357,#125358,#125359,#125360,#125361,#125362,#125363,
#125364,#125365,#125366,#125367,#125368,#125369,#125370,#125371,#125372,
#125373,#125374,#125375,#125376,#125377),.UNSPECIFIED.,.F.,.F.,(4,2,2,2,
2,2,2,2,2,2,2,2,2,4),(-0.729144904376339,-0.701294765627904,-0.644290240572763,
-0.584622721852303,-0.526155163852952,-0.468846061685899,-0.408761237620433,
-0.350964868034901,-0.292242330555774,-0.23291790866579,-0.175774000270549,
-0.116070886581869,-0.0573899304566333,0.),.UNSPECIFIED.) ;
#367=B_SPLINE_CURVE_WITH_KNOTS('',3,(#125385,#125386,#125387,#125388,#125389,
#125390,#125391,#125392,#125393,#125394,#125395,#125396,#125397,#125398,
#125399,#125400,#125401,#125402,#125403,#125404,#125405,#125406,#125407,
#125408,#125409,#125410,#125411,#125412,#125413,#125414),.UNSPECIFIED.,
 .F.,.F.,(4,2,2,2,2,2,2,2,2,2,2,2,2,2,4),(-8.55374923263164,-8.52045997548488,
-8.48812186400397,-8.43025873621608,-8.37009569721686,-8.31293715613035,
-8.25440154797182,-8.19477991623858,-8.1377605421172,-8.07858114325935,
-8.01975349658949,-7.96208993347597,-7.90214811438955,-7.84483111171218,
-7.79788942893258),.UNSPECIFIED.) ;
#368=B_SPLINE_CURVE_WITH_KNOTS('',3,(#125417,#125418,#125419,#125420,#125421,
#125422,#125423,#125424,#125425,#125426,#125427,#125428,#125429,#125430,
#125431,#125432,#125433,#125434,#125435,#125436,#125437,#125438,#125439,
#125440,#125441,#125442,#125443,#125444,#125445,#125446,#125447,#125448,
#125449,#125450,#125451,#125452),.UNSPECIFIED.,.F.,.F.,(4,2,2,2,2,2,2,2,
2,2,2,2,2,2,2,2,2,4),(-1.67472695159199,-1.63814253054756,-1.58112626326033,
-1.52144174075491,-1.46330248400391,-1.40546717323888,-1.34574854931093,
-1.28828093672951,-1.228494242623,-1.1695607477854,-1.11259684987605,-1.05293475628546,
-0.994649499089507,-0.937120115226852,-0.877236543088398,-0.819621249528116,
-0.760408371557094,-0.729144904376339),.UNSPECIFIED.) ;
#369=B_SPLINE_CURVE_WITH_KNOTS('',3,(#125454,#125455,#125456,#125457,#125458,
#125459,#125460,#125461,#125462,#125463,#125464,#125465,#125466,#125467,
#125468,#125469,#125470,#125471,#125472,#125473,#125474,#125475,#125476,
#125477,#125478,#125479,#125480,#125481,#125482,#125483,#125484,#125485,
#125486,#125487,#125488,#125489),.UNSPECIFIED.,.F.,.F.,(4,2,2,2,2,2,2,2,
2,2,2,2,2,2,2,2,2,4),(-7.79788942893258,-7.7864978331053,-7.72690027532479,
-7.66998381914493,-7.61100430828218,-7.55165262671408,-7.49415813115462,
-7.434404527004,-7.37683370109388,-7.31866970220167,-7.25906709251872,-7.20215576863061,
-7.14334343176941,-7.08339598828515,-7.02603560425023,-6.96643217276498,
-6.9085302919768,-6.85333016178901),.UNSPECIFIED.) ;
#370=B_SPLINE_CURVE_WITH_KNOTS('',3,(#125490,#125491,#125492,#125493,#125494,
#125495,#125496,#125497,#125498,#125499,#125500,#125501,#125502,#125503,
#125504,#125505,#125506,#125507,#125508,#125509,#125510,#125511,#125512,
#125513,#125514,#125515,#125516,#125517,#125518,#125519,#125520,#125521,
#125522,#125523,#125524,#125525),.UNSPECIFIED.,.F.,.F.,(4,2,2,2,2,2,2,2,
2,2,2,2,2,2,2,2,2,4),(-2.62073726926079,-2.57589168419096,-2.51862873581428,
-2.45854193473685,-2.40074535328825,-2.34210369906827,-2.28277616139501,
-2.22563231373495,-2.16594829107943,-2.10726356038932,-2.05010847618233,
-1.98978591242265,-1.93177619281583,-1.87350153298898,-1.81393494970357,
-1.75660268268265,-1.69693230395467,-1.67472695159199),.UNSPECIFIED.) ;
#371=B_SPLINE_CURVE_WITH_KNOTS('',3,(#125528,#125529,#125530,#125531,#125532,
#125533,#125534,#125535,#125536,#125537,#125538,#125539,#125540,#125541,
#125542,#125543,#125544,#125545,#125546,#125547,#125548,#125549),
 .UNSPECIFIED.,.F.,.F.,(4,2,2,2,2,2,2,2,2,2,4),(7.42653426035933,7.46701042314504,
7.51551605666961,7.56232997551886,7.61135461607121,7.65934114232017,7.70649931554284,
7.75579949517463,7.80323150261535,7.848007974901,7.89462988945302),
 .UNSPECIFIED.) ;
#372=B_SPLINE_CURVE_WITH_KNOTS('',3,(#125552,#125553,#125554,#125555,#125556,
#125557,#125558,#125559,#125560,#125561,#125562,#125563,#125564,#125565),
 .UNSPECIFIED.,.F.,.F.,(4,2,2,2,2,2,4),(9.99999999993084E-7,0.0454152741647829,
0.0934842511977,0.142483198960695,0.189312581462748,0.237893912869686,0.275540243682509),
 .UNSPECIFIED.) ;
#373=B_SPLINE_CURVE_WITH_KNOTS('',3,(#125585,#125586,#125587,#125588,#125589,
#125590,#125591,#125592,#125593,#125594,#125595,#125596,#125597,#125598,
#125599,#125600,#125601,#125602,#125603,#125604,#125605,#125606,#125607,
#125608,#125609,#125610,#125611,#125612,#125613,#125614),.UNSPECIFIED.,
 .F.,.F.,(4,2,2,2,2,2,2,2,2,2,2,2,2,2,4),(0.102793946330879,0.14065908540827,
0.207546049472987,0.277181081921595,0.341925843104979,0.425232051113792,
0.529553206832786,0.635138456761143,0.687061075445346,0.791098170318975,
0.901479157744014,1.02330053588931,1.15825935025609,1.22953088710868,1.29476085683451),
 .UNSPECIFIED.) ;
#374=B_SPLINE_CURVE_WITH_KNOTS('',3,(#125618,#125619,#125620,#125621,#125622,
#125623,#125624,#125625),.UNSPECIFIED.,.F.,.F.,(4,2,2,4),(0.,0.0368526993038302,
0.0772866279385214,0.102793946330879),.UNSPECIFIED.) ;
#375=B_SPLINE_CURVE_WITH_KNOTS('',3,(#125626,#125627,#125628,#125629,#125630,
#125631,#125632,#125633,#125634,#125635,#125636,#125637),.UNSPECIFIED.,
 .F.,.F.,(4,2,2,2,2,4),(-0.166237454912908,-0.14614759649084,-0.124790609402371,
-0.083627563805611,-0.0424146450456111,0.),.UNSPECIFIED.) ;
#376=B_SPLINE_CURVE_WITH_KNOTS('',3,(#126352,#126353,#126354,#126355,#126356,
#126357,#126358,#126359,#126360,#126361),.UNSPECIFIED.,.F.,.F.,(4,3,3,4),
(0.,8.73464104464917E-5,0.000174692824679549,0.000283410104056903),
 .UNSPECIFIED.) ;
#467=(
BOUNDED_SURFACE()
B_SPLINE_SURFACE(1,2,((#125809,#125810,#125811,#125812,#125813,#125814,
#125815,#125816,#125817,#125818,#125819,#125820,#125821,#125822,#125823,
#125824,#125825,#125826,#125827,#125828,#125829,#125830,#125831,#125832,
#125833,#125834,#125835,#125836,#125837,#125838,#125839,#125840,#125841,
#125842,#125843,#125844,#125845,#125846,#125847,#125848,#125849,#125850,
#125851,#125852,#125853,#125854,#125855,#125856,#125857,#125858,#125859,
#125860,#125861,#125862,#125863,#125864,#125865,#125866,#125867,#125868,
#125869,#125870,#125871,#125872,#125873,#125874,#125875,#125876,#125877,
#125878,#125879,#125880,#125881,#125882,#125883,#125884,#125885,#125886,
#125887,#125888,#125889,#125890,#125891,#125892,#125893,#125894,#125895,
#125896,#125897,#125898,#125899,#125900,#125901,#125902,#125903,#125904,
#125905,#125906,#125907,#125908,#125909,#125910,#125911,#125912,#125913,
#125914,#125915,#125916,#125917,#125918,#125919,#125920,#125921,#125922,
#125923,#125924,#125925,#125926,#125927,#125928,#125929,#125930,#125931,
#125932,#125933,#125934,#125935,#125936,#125937,#125938,#125939,#125940,
#125941,#125942,#125943),(#125944,#125945,#125946,#125947,#125948,#125949,
#125950,#125951,#125952,#125953,#125954,#125955,#125956,#125957,#125958,
#125959,#125960,#125961,#125962,#125963,#125964,#125965,#125966,#125967,
#125968,#125969,#125970,#125971,#125972,#125973,#125974,#125975,#125976,
#125977,#125978,#125979,#125980,#125981,#125982,#125983,#125984,#125985,
#125986,#125987,#125988,#125989,#125990,#125991,#125992,#125993,#125994,
#125995,#125996,#125997,#125998,#125999,#126000,#126001,#126002,#126003,
#126004,#126005,#126006,#126007,#126008,#126009,#126010,#126011,#126012,
#126013,#126014,#126015,#126016,#126017,#126018,#126019,#126020,#126021,
#126022,#126023,#126024,#126025,#126026,#126027,#126028,#126029,#126030,
#126031,#126032,#126033,#126034,#126035,#126036,#126037,#126038,#126039,
#126040,#126041,#126042,#126043,#126044,#126045,#126046,#126047,#126048,
#126049,#126050,#126051,#126052,#126053,#126054,#126055,#126056,#126057,
#126058,#126059,#126060,#126061,#126062,#126063,#126064,#126065,#126066,
#126067,#126068,#126069,#126070,#126071,#126072,#126073,#126074,#126075,
#126076,#126077,#126078)),.UNSPECIFIED.,.F.,.F.,.F.)
B_SPLINE_SURFACE_WITH_KNOTS((2,2),(3,2,2,2,2,2,2,2,2,2,2,2,2,2,2,2,2,2,
2,2,2,2,2,2,2,2,2,2,2,2,2,2,2,2,2,2,2,2,2,2,2,2,2,2,2,2,2,2,2,2,2,2,2,2,
2,2,2,2,2,2,2,2,2,2,2,2,2,3),(0.,1.00006111776867),(0.,0.0138888888888889,
0.0277777777777778,0.0416666666666667,0.0555555555555556,0.0694444444444444,
0.0833333333333333,0.0972222222222222,0.111111111111111,0.125,0.138888888888889,
0.152777777777778,0.166666666666667,0.180555555555556,0.194444444444444,
0.208333333333333,0.222222222222222,0.236111111111111,0.25,0.263888888888889,
0.277777777777778,0.291666666666667,0.305555555555556,0.319444444444444,
0.333333333333333,0.347222222222222,0.361111111111111,0.375,0.388888888888889,
0.402777777777778,0.416666666666667,0.430555555555556,0.444444444444444,
0.458333333333333,0.472222222222222,0.486111111111111,0.5,0.513888888888889,
0.527777777777778,0.541666666666667,0.555555555555556,0.569444444444444,
0.583333333333333,0.597222222222222,0.611111111111111,0.625,0.638888888888889,
0.652777777777778,0.666666666666667,0.680555555555556,0.694444444444444,
0.708333333333333,0.722222222222222,0.736111111111111,0.75,0.763888888888889,
0.777777777777778,0.791666666666667,0.805555555555556,0.819444444444444,
0.833333333333333,0.847222222222222,0.861111111111111,0.875,0.888888888888889,
0.902777777777778,0.916666666666667,0.920887586444199),.UNSPECIFIED.)
GEOMETRIC_REPRESENTATION_ITEM()
RATIONAL_B_SPLINE_SURFACE(((1.,0.866025403784439,1.,0.866025403784439,1.,
0.866025403784439,1.,0.866025403784439,1.,0.866025403784439,1.,0.866025403784439,
1.,0.866025403784439,1.,0.866025403784439,1.,0.866025403784439,1.,0.866025403784439,
1.,0.866025403784439,1.,0.866025403784439,1.,0.866025403784439,1.,0.866025403784439,
1.,0.866025403784439,1.,0.866025403784439,1.,0.866025403784439,1.,0.866025403784439,
1.,0.866025403784439,1.,0.866025403784439,1.,0.866025403784439,1.,0.866025403784439,
1.,0.866025403784439,1.,0.866025403784439,1.,0.866025403784439,1.,0.866025403784439,
1.,0.866025403784439,1.,0.866025403784439,1.,0.866025403784439,1.,0.866025403784439,
1.,0.866025403784439,1.,0.866025403784439,1.,0.866025403784439,1.,0.866025403784439,
1.,0.866025403784439,1.,0.866025403784439,1.,0.866025403784439,1.,0.866025403784439,
1.,0.866025403784439,1.,0.866025403784439,1.,0.866025403784439,1.,0.866025403784439,
1.,0.866025403784439,1.,0.866025403784439,1.,0.866025403784439,1.,0.866025403784439,
1.,0.866025403784439,1.,0.866025403784439,1.,0.866025403784439,1.,0.866025403784439,
1.,0.866025403784439,1.,0.866025403784439,1.,0.866025403784439,1.,0.866025403784439,
1.,0.866025403784439,1.,0.866025403784439,1.,0.866025403784439,1.,0.866025403784439,
1.,0.866025403784439,1.,0.866025403784439,1.,0.866025403784439,1.,0.866025403784439,
1.,0.866025403784439,1.,0.866025403784439,1.,0.866025403784439,1.,0.866025403784439,
1.,0.959284286354576,0.943316090290602),(1.,0.866025403784439,1.,0.866025403784439,
1.,0.866025403784439,1.,0.866025403784439,1.,0.866025403784439,1.,0.866025403784439,
1.,0.866025403784439,1.,0.866025403784439,1.,0.866025403784439,1.,0.866025403784439,
1.,0.866025403784439,1.,0.866025403784439,1.,0.866025403784439,1.,0.866025403784439,
1.,0.866025403784439,1.,0.866025403784439,1.,0.866025403784439,1.,0.866025403784439,
1.,0.866025403784439,1.,0.866025403784439,1.,0.866025403784439,1.,0.866025403784439,
1.,0.866025403784439,1.,0.866025403784439,1.,0.866025403784439,1.,0.866025403784439,
1.,0.866025403784439,1.,0.866025403784439,1.,0.866025403784439,1.,0.866025403784439,
1.,0.866025403784439,1.,0.866025403784439,1.,0.866025403784439,1.,0.866025403784439,
1.,0.866025403784439,1.,0.866025403784439,1.,0.866025403784439,1.,0.866025403784439,
1.,0.866025403784439,1.,0.866025403784439,1.,0.866025403784439,1.,0.866025403784439,
1.,0.866025403784439,1.,0.866025403784439,1.,0.866025403784439,1.,0.866025403784439,
1.,0.866025403784439,1.,0.866025403784439,1.,0.866025403784439,1.,0.866025403784439,
1.,0.866025403784439,1.,0.866025403784439,1.,0.866025403784439,1.,0.866025403784439,
1.,0.866025403784439,1.,0.866025403784439,1.,0.866025403784439,1.,0.866025403784439,
1.,0.866025403784439,1.,0.866025403784439,1.,0.866025403784439,1.,0.866025403784439,
1.,0.866025403784439,1.,0.866025403784439,1.,0.866025403784439,1.,0.866025403784439,
1.,0.959284286354576,0.943316090290602)))
REPRESENTATION_ITEM('')
SURFACE()
) ;
#468=(
BOUNDED_SURFACE()
B_SPLINE_SURFACE(1,2,((#126080,#126081,#126082,#126083,#126084,#126085,
#126086,#126087,#126088,#126089,#126090,#126091,#126092,#126093,#126094,
#126095,#126096,#126097,#126098,#126099,#126100,#126101,#126102,#126103,
#126104,#126105,#126106,#126107,#126108,#126109,#126110,#126111,#126112,
#126113,#126114,#126115,#126116,#126117,#126118,#126119,#126120,#126121,
#126122,#126123,#126124,#126125,#126126,#126127,#126128,#126129,#126130,
#126131,#126132,#126133,#126134,#126135,#126136,#126137,#126138,#126139,
#126140,#126141,#126142,#126143,#126144,#126145,#126146,#126147,#126148,
#126149,#126150,#126151,#126152,#126153,#126154,#126155,#126156,#126157,
#126158,#126159,#126160,#126161,#126162,#126163,#126164,#126165,#126166,
#126167,#126168,#126169,#126170,#126171,#126172,#126173,#126174,#126175,
#126176,#126177,#126178,#126179,#126180,#126181,#126182,#126183,#126184,
#126185,#126186,#126187,#126188,#126189,#126190,#126191,#126192,#126193,
#126194,#126195,#126196,#126197,#126198,#126199,#126200,#126201,#126202,
#126203,#126204,#126205,#126206,#126207,#126208,#126209,#126210,#126211,
#126212,#126213,#126214),(#126215,#126216,#126217,#126218,#126219,#126220,
#126221,#126222,#126223,#126224,#126225,#126226,#126227,#126228,#126229,
#126230,#126231,#126232,#126233,#126234,#126235,#126236,#126237,#126238,
#126239,#126240,#126241,#126242,#126243,#126244,#126245,#126246,#126247,
#126248,#126249,#126250,#126251,#126252,#126253,#126254,#126255,#126256,
#126257,#126258,#126259,#126260,#126261,#126262,#126263,#126264,#126265,
#126266,#126267,#126268,#126269,#126270,#126271,#126272,#126273,#126274,
#126275,#126276,#126277,#126278,#126279,#126280,#126281,#126282,#126283,
#126284,#126285,#126286,#126287,#126288,#126289,#126290,#126291,#126292,
#126293,#126294,#126295,#126296,#126297,#126298,#126299,#126300,#126301,
#126302,#126303,#126304,#126305,#126306,#126307,#126308,#126309,#126310,
#126311,#126312,#126313,#126314,#126315,#126316,#126317,#126318,#126319,
#126320,#126321,#126322,#126323,#126324,#126325,#126326,#126327,#126328,
#126329,#126330,#126331,#126332,#126333,#126334,#126335,#126336,#126337,
#126338,#126339,#126340,#126341,#126342,#126343,#126344,#126345,#126346,
#126347,#126348,#126349)),.UNSPECIFIED.,.F.,.F.,.F.)
B_SPLINE_SURFACE_WITH_KNOTS((2,2),(3,2,2,2,2,2,2,2,2,2,2,2,2,2,2,2,2,2,
2,2,2,2,2,2,2,2,2,2,2,2,2,2,2,2,2,2,2,2,2,2,2,2,2,2,2,2,2,2,2,2,2,2,2,2,
2,2,2,2,2,2,2,2,2,2,2,2,2,3),(0.,1.),(0.,0.0138888888888889,0.0277777777777778,
0.0416666666666667,0.0555555555555556,0.0694444444444444,0.0833333333333333,
0.0972222222222222,0.111111111111111,0.125,0.138888888888889,0.152777777777778,
0.166666666666667,0.180555555555556,0.194444444444444,0.208333333333333,
0.222222222222222,0.236111111111111,0.25,0.263888888888889,0.277777777777778,
0.291666666666667,0.305555555555556,0.319444444444444,0.333333333333333,
0.347222222222222,0.361111111111111,0.375,0.388888888888889,0.402777777777778,
0.416666666666667,0.430555555555556,0.444444444444444,0.458333333333333,
0.472222222222222,0.486111111111111,0.5,0.513888888888889,0.527777777777778,
0.541666666666667,0.555555555555556,0.569444444444444,0.583333333333333,
0.597222222222222,0.611111111111111,0.625,0.638888888888889,0.652777777777778,
0.666666666666667,0.680555555555556,0.694444444444444,0.708333333333333,
0.722222222222222,0.736111111111111,0.75,0.763888888888889,0.777777777777778,
0.791666666666667,0.805555555555556,0.819444444444444,0.833333333333333,
0.847222222222222,0.861111111111111,0.875,0.888888888888889,0.902777777777778,
0.916666666666667,0.920887434615967),.UNSPECIFIED.)
GEOMETRIC_REPRESENTATION_ITEM()
RATIONAL_B_SPLINE_SURFACE(((1.,0.866025403784439,1.,0.866025403784439,1.,
0.866025403784439,1.,0.866025403784439,1.,0.866025403784439,1.,0.866025403784439,
1.,0.866025403784439,1.,0.866025403784439,1.,0.866025403784439,1.,0.866025403784439,
1.,0.866025403784439,1.,0.866025403784439,1.,0.866025403784439,1.,0.866025403784439,
1.,0.866025403784439,1.,0.866025403784439,1.,0.866025403784439,1.,0.866025403784439,
1.,0.866025403784439,1.,0.866025403784439,1.,0.866025403784439,1.,0.866025403784439,
1.,0.866025403784439,1.,0.866025403784439,1.,0.866025403784439,1.,0.866025403784439,
1.,0.866025403784439,1.,0.866025403784439,1.,0.866025403784439,1.,0.866025403784439,
1.,0.866025403784439,1.,0.866025403784439,1.,0.866025403784439,1.,0.866025403784439,
1.,0.866025403784439,1.,0.866025403784439,1.,0.866025403784439,1.,0.866025403784439,
1.,0.866025403784439,1.,0.866025403784439,1.,0.866025403784439,1.,0.866025403784439,
1.,0.866025403784439,1.,0.866025403784439,1.,0.866025403784439,1.,0.866025403784439,
1.,0.866025403784439,1.,0.866025403784439,1.,0.866025403784439,1.,0.866025403784439,
1.,0.866025403784439,1.,0.866025403784439,1.,0.866025403784439,1.,0.866025403784439,
1.,0.866025403784439,1.,0.866025403784439,1.,0.866025403784439,1.,0.866025403784439,
1.,0.866025403784439,1.,0.866025403784439,1.,0.866025403784439,1.,0.866025403784439,
1.,0.866025403784439,1.,0.866025403784439,1.,0.866025403784439,1.,0.866025403784439,
1.,0.959285750915652,0.943317239087869),(1.,0.866025403784439,1.,0.866025403784439,
1.,0.866025403784439,1.,0.866025403784439,1.,0.866025403784439,1.,0.866025403784439,
1.,0.866025403784439,1.,0.866025403784439,1.,0.866025403784439,1.,0.866025403784439,
1.,0.866025403784439,1.,0.866025403784439,1.,0.866025403784439,1.,0.866025403784439,
1.,0.866025403784439,1.,0.866025403784439,1.,0.866025403784439,1.,0.866025403784439,
1.,0.866025403784439,1.,0.866025403784439,1.,0.866025403784439,1.,0.866025403784439,
1.,0.866025403784439,1.,0.866025403784439,1.,0.866025403784439,1.,0.866025403784439,
1.,0.866025403784439,1.,0.866025403784439,1.,0.866025403784439,1.,0.866025403784439,
1.,0.866025403784439,1.,0.866025403784439,1.,0.866025403784439,1.,0.866025403784439,
1.,0.866025403784439,1.,0.866025403784439,1.,0.866025403784439,1.,0.866025403784439,
1.,0.866025403784439,1.,0.866025403784439,1.,0.866025403784439,1.,0.866025403784439,
1.,0.866025403784439,1.,0.866025403784439,1.,0.866025403784439,1.,0.866025403784439,
1.,0.866025403784439,1.,0.866025403784439,1.,0.866025403784439,1.,0.866025403784439,
1.,0.866025403784439,1.,0.866025403784439,1.,0.866025403784439,1.,0.866025403784439,
1.,0.866025403784439,1.,0.866025403784439,1.,0.866025403784439,1.,0.866025403784439,
1.,0.866025403784439,1.,0.866025403784439,1.,0.866025403784439,1.,0.866025403784439,
1.,0.866025403784439,1.,0.866025403784439,1.,0.866025403784439,1.,0.866025403784439,
1.,0.959285750915652,0.943317239087869)))
REPRESENTATION_ITEM('')
SURFACE()
) ;
#473=SHAPE_REPRESENTATION_RELATIONSHIP('SRR','None',#126603,#479) ;
#479=ADVANCED_BREP_SHAPE_REPRESENTATION('',(#4180),#126569) ;
#4170=STYLED_ITEM('',(#126644),#4180) ;
#4180=MANIFOLD_SOLID_BREP('Body1',#67694) ;
#4983=ELLIPSE('',#76691,1.73204548364451,1.5) ;
#4984=ELLIPSE('',#76692,1.73205681329418,1.5) ;
#5061=FACE_BOUND('',#24666,.T.) ;
#5062=FACE_BOUND('',#24668,.T.) ;
#5913=PLANE('',#76749) ;
#5914=PLANE('',#76750) ;
#5915=PLANE('',#76751) ;
#5916=PLANE('',#76752) ;
#5917=PLANE('',#76753) ;
#5918=PLANE('',#76754) ;
#5919=PLANE('',#76755) ;
#5920=PLANE('',#76756) ;
#5921=PLANE('',#76757) ;
#5922=PLANE('',#76759) ;
#5923=PLANE('',#76760) ;
#5924=PLANE('',#76761) ;
#7866=CYLINDRICAL_SURFACE('',#76670,1.2293670625) ;
#7867=CYLINDRICAL_SURFACE('',#76671,1.2293670625) ;
#7868=CYLINDRICAL_SURFACE('',#76672,1.2293670625) ;
#7869=CYLINDRICAL_SURFACE('',#76673,1.2293670625) ;
#7870=CYLINDRICAL_SURFACE('',#76674,1.2293670625) ;
#7871=CYLINDRICAL_SURFACE('',#76675,1.2293670625) ;
#7872=CYLINDRICAL_SURFACE('',#76676,1.2293670625) ;
#7873=CYLINDRICAL_SURFACE('',#76677,1.2293670625) ;
#7874=CYLINDRICAL_SURFACE('',#76678,1.2293670625) ;
#7875=CYLINDRICAL_SURFACE('',#76679,1.2293670625) ;
#7876=CYLINDRICAL_SURFACE('',#76680,1.5) ;
#7877=CYLINDRICAL_SURFACE('',#76682,1.5) ;
#7878=CYLINDRICAL_SURFACE('',#76683,1.5) ;
#7879=CYLINDRICAL_SURFACE('',#76684,1.5) ;
#7880=CYLINDRICAL_SURFACE('',#76685,1.5) ;
#7881=CYLINDRICAL_SURFACE('',#76686,1.5) ;
#7882=CYLINDRICAL_SURFACE('',#76687,1.5) ;
#7883=CYLINDRICAL_SURFACE('',#76688,1.5) ;
#7884=CYLINDRICAL_SURFACE('',#76689,1.5) ;
#7885=CYLINDRICAL_SURFACE('',#76693,1.5) ;
#7886=CYLINDRICAL_SURFACE('',#76694,1.2293670625) ;
#7887=CYLINDRICAL_SURFACE('',#76699,1.25) ;
#7888=CYLINDRICAL_SURFACE('',#76707,2.49807621135332) ;
#7889=CYLINDRICAL_SURFACE('',#76710,2.49807621135332) ;
#7890=CYLINDRICAL_SURFACE('',#76713,2.49807621135332) ;
#7891=CYLINDRICAL_SURFACE('',#76716,2.49807621135332) ;
#7892=CYLINDRICAL_SURFACE('',#76719,2.49807621135332) ;
#7893=CYLINDRICAL_SURFACE('',#76722,2.49807621135332) ;
#11944=LINE('',#124045,#16060) ;
#11945=LINE('',#124068,#16061) ;
#11946=LINE('',#124092,#16062) ;
#11947=LINE('',#124172,#16063) ;
#11948=LINE('',#124248,#16064) ;
#11949=LINE('',#124324,#16065) ;
#11950=LINE('',#124400,#16066) ;
#11951=LINE('',#124476,#16067) ;
#11952=LINE('',#124552,#16068) ;
#11953=LINE('',#124628,#16069) ;
#11954=LINE('',#124708,#16070) ;
#11955=LINE('',#124784,#16071) ;
#11956=LINE('',#124811,#16072) ;
#11957=LINE('',#124887,#16073) ;
#11958=LINE('',#124963,#16074) ;
#11959=LINE('',#125039,#16075) ;
#11960=LINE('',#125115,#16076) ;
#11961=LINE('',#125191,#16077) ;
#11962=LINE('',#125269,#16078) ;
#11963=LINE('',#125348,#16079) ;
#11964=LINE('',#125381,#16080) ;
#11965=LINE('',#125416,#16081) ;
#11966=LINE('',#125570,#16082) ;
#11967=LINE('',#125575,#16083) ;
#11968=LINE('',#125578,#16084) ;
#11969=LINE('',#125616,#16085) ;
#11970=LINE('',#125641,#16086) ;
#11971=LINE('',#125645,#16087) ;
#11972=LINE('',#125650,#16088) ;
#11973=LINE('',#125654,#16089) ;
#11974=LINE('',#125659,#16090) ;
#11975=LINE('',#125663,#16091) ;
#11976=LINE('',#125668,#16092) ;
#11977=LINE('',#125672,#16093) ;
#11978=LINE('',#125677,#16094) ;
#11979=LINE('',#125681,#16095) ;
#11980=LINE('',#125686,#16096) ;
#11981=LINE('',#125690,#16097) ;
#11982=LINE('',#126079,#16098) ;
#11983=LINE('',#126363,#16099) ;
#11984=LINE('',#126365,#16100) ;
#16060=VECTOR('',#98716,1.2293670625) ;
#16061=VECTOR('',#98717,10.) ;
#16062=VECTOR('',#98720,1.2293670625) ;
#16063=VECTOR('',#98723,1.2293670625) ;
#16064=VECTOR('',#98726,1.2293670625) ;
#16065=VECTOR('',#98729,1.2293670625) ;
#16066=VECTOR('',#98732,1.2293670625) ;
#16067=VECTOR('',#98735,1.2293670625) ;
#16068=VECTOR('',#98738,1.2293670625) ;
#16069=VECTOR('',#98741,1.2293670625) ;
#16070=VECTOR('',#98744,1.2293670625) ;
#16071=VECTOR('',#98747,1.5) ;
#16072=VECTOR('',#98752,1.5) ;
#16073=VECTOR('',#98755,1.5) ;
#16074=VECTOR('',#98758,1.5) ;
#16075=VECTOR('',#98761,1.5) ;
#16076=VECTOR('',#98764,1.5) ;
#16077=VECTOR('',#98767,1.5) ;
#16078=VECTOR('',#98770,1.5) ;
#16079=VECTOR('',#98775,1.5) ;
#16080=VECTOR('',#98778,10.) ;
#16081=VECTOR('',#98781,1.5) ;
#16082=VECTOR('',#98792,1.6) ;
#16083=VECTOR('',#98799,1.25) ;
#16084=VECTOR('',#98802,1.25) ;
#16085=VECTOR('',#98811,0.999999999999998) ;
#16086=VECTOR('',#98816,1000.) ;
#16087=VECTOR('',#98819,1000.) ;
#16088=VECTOR('',#98824,1000.) ;
#16089=VECTOR('',#98827,1000.) ;
#16090=VECTOR('',#98832,1000.) ;
#16091=VECTOR('',#98835,1000.) ;
#16092=VECTOR('',#98840,1000.) ;
#16093=VECTOR('',#98843,1000.) ;
#16094=VECTOR('',#98848,1000.) ;
#16095=VECTOR('',#98851,1000.) ;
#16096=VECTOR('',#98856,1000.) ;
#16097=VECTOR('',#98859,1000.) ;
#16098=VECTOR('',#98928,10.) ;
#16099=VECTOR('',#98933,1000.) ;
#16100=VECTOR('',#98936,1000.) ;
#16135=CONICAL_SURFACE('',#76696,1.6,0.785398163397445) ;
#16136=CONICAL_SURFACE('',#76701,1.25,1.02974425867665) ;
#16137=CONICAL_SURFACE('',#76705,0.999999999999998,0.785398163397446) ;
#16138=CONICAL_SURFACE('',#76725,2.49807621135332,0.785398163397447) ;
#16139=CONICAL_SURFACE('',#76727,2.49807621135332,0.785398163397447) ;
#16140=CONICAL_SURFACE('',#76729,2.49807621135332,0.785398163397447) ;
#16141=CONICAL_SURFACE('',#76731,2.49807621135332,0.785398163397447) ;
#16142=CONICAL_SURFACE('',#76733,2.49807621135332,0.785398163397447) ;
#16143=CONICAL_SURFACE('',#76735,2.49807621135332,0.785398163397447) ;
#16144=CONICAL_SURFACE('',#76737,2.25,0.785398163397443) ;
#16145=CONICAL_SURFACE('',#76739,2.25,0.785398163397443) ;
#16146=CONICAL_SURFACE('',#76741,2.25,0.785398163397443) ;
#16147=CONICAL_SURFACE('',#76743,2.25,0.785398163397443) ;
#16148=CONICAL_SURFACE('',#76745,2.25,0.785398163397443) ;
#16149=CONICAL_SURFACE('',#76747,2.25,0.785398163397443) ;
#20307=FACE_OUTER_BOUND('',#24621,.T.) ;
#20308=FACE_OUTER_BOUND('',#24622,.T.) ;
#20309=FACE_OUTER_BOUND('',#24623,.T.) ;
#20310=FACE_OUTER_BOUND('',#24624,.T.) ;
#20311=FACE_OUTER_BOUND('',#24625,.T.) ;
#20312=FACE_OUTER_BOUND('',#24626,.T.) ;
#20313=FACE_OUTER_BOUND('',#24627,.T.) ;
#20314=FACE_OUTER_BOUND('',#24628,.T.) ;
#20315=FACE_OUTER_BOUND('',#24629,.T.) ;
#20316=FACE_OUTER_BOUND('',#24630,.T.) ;
#20317=FACE_OUTER_BOUND('',#24631,.T.) ;
#20318=FACE_OUTER_BOUND('',#24632,.T.) ;
#20319=FACE_OUTER_BOUND('',#24633,.T.) ;
#20320=FACE_OUTER_BOUND('',#24634,.T.) ;
#20321=FACE_OUTER_BOUND('',#24635,.T.) ;
#20322=FACE_OUTER_BOUND('',#24636,.T.) ;
#20323=FACE_OUTER_BOUND('',#24637,.T.) ;
#20324=FACE_OUTER_BOUND('',#24638,.T.) ;
#20325=FACE_OUTER_BOUND('',#24639,.T.) ;
#20326=FACE_OUTER_BOUND('',#24640,.T.) ;
#20327=FACE_OUTER_BOUND('',#24641,.T.) ;
#20328=FACE_OUTER_BOUND('',#24642,.T.) ;
#20329=FACE_OUTER_BOUND('',#24643,.T.) ;
#20330=FACE_OUTER_BOUND('',#24644,.T.) ;
#20331=FACE_OUTER_BOUND('',#24645,.T.) ;
#20332=FACE_OUTER_BOUND('',#24646,.T.) ;
#20333=FACE_OUTER_BOUND('',#24647,.T.) ;
#20334=FACE_OUTER_BOUND('',#24648,.T.) ;
#20335=FACE_OUTER_BOUND('',#24649,.T.) ;
#20336=FACE_OUTER_BOUND('',#24650,.T.) ;
#20337=FACE_OUTER_BOUND('',#24651,.T.) ;
#20338=FACE_OUTER_BOUND('',#24652,.T.) ;
#20339=FACE_OUTER_BOUND('',#24653,.T.) ;
#20340=FACE_OUTER_BOUND('',#24654,.T.) ;
#20341=FACE_OUTER_BOUND('',#24655,.T.) ;
#20342=FACE_OUTER_BOUND('',#24656,.T.) ;
#20343=FACE_OUTER_BOUND('',#24657,.T.) ;
#20344=FACE_OUTER_BOUND('',#24658,.T.) ;
#20345=FACE_OUTER_BOUND('',#24659,.T.) ;
#20346=FACE_OUTER_BOUND('',#24660,.T.) ;
#20347=FACE_OUTER_BOUND('',#24661,.T.) ;
#20348=FACE_OUTER_BOUND('',#24662,.T.) ;
#20349=FACE_OUTER_BOUND('',#24663,.T.) ;
#20350=FACE_OUTER_BOUND('',#24664,.T.) ;
#20351=FACE_OUTER_BOUND('',#24665,.T.) ;
#20352=FACE_OUTER_BOUND('',#24667,.T.) ;
#20353=FACE_OUTER_BOUND('',#24669,.T.) ;
#20354=FACE_OUTER_BOUND('',#24670,.T.) ;
#20355=FACE_OUTER_BOUND('',#24671,.T.) ;
#20356=FACE_OUTER_BOUND('',#24672,.T.) ;
#20357=FACE_OUTER_BOUND('',#24673,.T.) ;
#20358=FACE_OUTER_BOUND('',#24674,.T.) ;
#20359=FACE_OUTER_BOUND('',#24675,.T.) ;
#20360=FACE_OUTER_BOUND('',#24676,.T.) ;
#20361=FACE_OUTER_BOUND('',#24677,.T.) ;
#20362=FACE_OUTER_BOUND('',#24678,.T.) ;
#20363=FACE_OUTER_BOUND('',#24679,.T.) ;
#20364=FACE_OUTER_BOUND('',#24680,.T.) ;
#24621=EDGE_LOOP('',(#62358,#62359,#62360,#62361)) ;
#24622=EDGE_LOOP('',(#62362,#62363,#62364,#62365)) ;
#24623=EDGE_LOOP('',(#62366,#62367,#62368,#62369)) ;
#24624=EDGE_LOOP('',(#62370,#62371,#62372,#62373)) ;
#24625=EDGE_LOOP('',(#62374,#62375,#62376,#62377)) ;
#24626=EDGE_LOOP('',(#62378,#62379,#62380,#62381)) ;
#24627=EDGE_LOOP('',(#62382,#62383,#62384,#62385)) ;
#24628=EDGE_LOOP('',(#62386,#62387,#62388,#62389)) ;
#24629=EDGE_LOOP('',(#62390,#62391,#62392,#62393)) ;
#24630=EDGE_LOOP('',(#62394,#62395,#62396,#62397)) ;
#24631=EDGE_LOOP('',(#62398,#62399,#62400,#62401)) ;
#24632=EDGE_LOOP('',(#62402,#62403,#62404,#62405)) ;
#24633=EDGE_LOOP('',(#62406,#62407,#62408,#62409)) ;
#24634=EDGE_LOOP('',(#62410,#62411,#62412,#62413)) ;
#24635=EDGE_LOOP('',(#62414,#62415,#62416,#62417)) ;
#24636=EDGE_LOOP('',(#62418,#62419,#62420,#62421)) ;
#24637=EDGE_LOOP('',(#62422,#62423,#62424,#62425)) ;
#24638=EDGE_LOOP('',(#62426,#62427,#62428,#62429)) ;
#24639=EDGE_LOOP('',(#62430,#62431,#62432,#62433,#62434,#62435,#62436,#62437,
#62438,#62439)) ;
#24640=EDGE_LOOP('',(#62440,#62441,#62442,#62443)) ;
#24641=EDGE_LOOP('',(#62444,#62445,#62446,#62447)) ;
#24642=EDGE_LOOP('',(#62448,#62449,#62450,#62451)) ;
#24643=EDGE_LOOP('',(#62452,#62453,#62454,#62455)) ;
#24644=EDGE_LOOP('',(#62456,#62457,#62458)) ;
#24645=EDGE_LOOP('',(#62459,#62460,#62461,#62462)) ;
#24646=EDGE_LOOP('',(#62463,#62464,#62465,#62466,#62467,#62468,#62469,#62470)) ;
#24647=EDGE_LOOP('',(#62471,#62472,#62473,#62474)) ;
#24648=EDGE_LOOP('',(#62475,#62476,#62477,#62478)) ;
#24649=EDGE_LOOP('',(#62479,#62480,#62481,#62482)) ;
#24650=EDGE_LOOP('',(#62483,#62484,#62485,#62486)) ;
#24651=EDGE_LOOP('',(#62487,#62488,#62489,#62490)) ;
#24652=EDGE_LOOP('',(#62491,#62492,#62493,#62494)) ;
#24653=EDGE_LOOP('',(#62495,#62496,#62497,#62498)) ;
#24654=EDGE_LOOP('',(#62499,#62500,#62501,#62502)) ;
#24655=EDGE_LOOP('',(#62503,#62504,#62505,#62506)) ;
#24656=EDGE_LOOP('',(#62507,#62508,#62509,#62510)) ;
#24657=EDGE_LOOP('',(#62511,#62512,#62513,#62514)) ;
#24658=EDGE_LOOP('',(#62515,#62516,#62517,#62518)) ;
#24659=EDGE_LOOP('',(#62519,#62520,#62521,#62522)) ;
#24660=EDGE_LOOP('',(#62523,#62524,#62525,#62526)) ;
#24661=EDGE_LOOP('',(#62527,#62528,#62529,#62530)) ;
#24662=EDGE_LOOP('',(#62531,#62532,#62533,#62534)) ;
#24663=EDGE_LOOP('',(#62535,#62536,#62537,#62538)) ;
#24664=EDGE_LOOP('',(#62539,#62540,#62541,#62542)) ;
#24665=EDGE_LOOP('',(#62543,#62544,#62545,#62546,#62547,#62548)) ;
#24666=EDGE_LOOP('',(#62549)) ;
#24667=EDGE_LOOP('',(#62550,#62551,#62552,#62553,#62554,#62555)) ;
#24668=EDGE_LOOP('',(#62556)) ;
#24669=EDGE_LOOP('',(#62557)) ;
#24670=EDGE_LOOP('',(#62558,#62559,#62560,#62561,#62562,#62563)) ;
#24671=EDGE_LOOP('',(#62564,#62565,#62566,#62567,#62568,#62569)) ;
#24672=EDGE_LOOP('',(#62570,#62571,#62572,#62573,#62574,#62575)) ;
#24673=EDGE_LOOP('',(#62576,#62577,#62578,#62579,#62580,#62581)) ;
#24674=EDGE_LOOP('',(#62582,#62583,#62584,#62585,#62586,#62587)) ;
#24675=EDGE_LOOP('',(#62588,#62589,#62590,#62591,#62592,#62593)) ;
#24676=EDGE_LOOP('',(#62594,#62595,#62596,#62597,#62598,#62599,#62600,#62601,
#62602,#62603,#62604,#62605,#62606,#62607,#62608,#62609,#62610,#62611,#62612,
#62613,#62614,#62615,#62616,#62617)) ;
#24677=EDGE_LOOP('',(#62618,#62619,#62620,#62621,#62622,#62623,#62624,#62625,
#62626,#62627,#62628,#62629,#62630,#62631,#62632,#62633,#62634,#62635,#62636,
#62637,#62638,#62639,#62640,#62641,#62642)) ;
#24678=EDGE_LOOP('',(#62643,#62644,#62645)) ;
#24679=EDGE_LOOP('',(#62646,#62647,#62648,#62649)) ;
#24680=EDGE_LOOP('',(#62650,#62651,#62652,#62653)) ;
#29419=CIRCLE('',#76681,1.5) ;
#29420=CIRCLE('',#76690,1.5) ;
#29421=CIRCLE('',#76695,1.22936706250017) ;
#29422=CIRCLE('',#76697,1.25) ;
#29423=CIRCLE('',#76698,1.6) ;
#29424=CIRCLE('',#76700,1.25) ;
#29425=CIRCLE('',#76703,1.6) ;
#29426=CIRCLE('',#76704,0.1) ;
#29427=CIRCLE('',#76706,0.999999999999998) ;
#29428=CIRCLE('',#76708,2.49807621135332) ;
#29429=CIRCLE('',#76709,2.49807621135332) ;
#29430=CIRCLE('',#76711,2.49807621135332) ;
#29431=CIRCLE('',#76712,2.49807621135332) ;
#29432=CIRCLE('',#76714,2.49807621135332) ;
#29433=CIRCLE('',#76715,2.49807621135332) ;
#29434=CIRCLE('',#76717,2.49807621135332) ;
#29435=CIRCLE('',#76718,2.49807621135332) ;
#29436=CIRCLE('',#76720,2.49807621135332) ;
#29437=CIRCLE('',#76721,2.49807621135332) ;
#29438=CIRCLE('',#76723,2.49807621135332) ;
#29439=CIRCLE('',#76724,2.49807621135332) ;
#29440=CIRCLE('',#76726,2.25) ;
#29441=CIRCLE('',#76728,2.25) ;
#29442=CIRCLE('',#76730,2.25) ;
#29443=CIRCLE('',#76732,2.25) ;
#29444=CIRCLE('',#76734,2.25) ;
#29445=CIRCLE('',#76736,2.25) ;
#29446=CIRCLE('',#76738,2.25) ;
#29447=CIRCLE('',#76740,2.25) ;
#29448=CIRCLE('',#76742,2.25) ;
#29449=CIRCLE('',#76744,2.25) ;
#29450=CIRCLE('',#76746,2.25) ;
#29451=CIRCLE('',#76748,2.25) ;
#29452=CIRCLE('',#76758,2.37313871770562) ;
#34550=VERTEX_POINT('',#124043) ;
#34551=VERTEX_POINT('',#124044) ;
#34552=VERTEX_POINT('',#124046) ;
#34553=VERTEX_POINT('',#124067) ;
#34554=VERTEX_POINT('',#124090) ;
#34555=VERTEX_POINT('',#124091) ;
#34556=VERTEX_POINT('',#124170) ;
#34557=VERTEX_POINT('',#124171) ;
#34558=VERTEX_POINT('',#124246) ;
#34559=VERTEX_POINT('',#124247) ;
#34560=VERTEX_POINT('',#124322) ;
#34561=VERTEX_POINT('',#124323) ;
#34562=VERTEX_POINT('',#124398) ;
#34563=VERTEX_POINT('',#124399) ;
#34564=VERTEX_POINT('',#124474) ;
#34565=VERTEX_POINT('',#124475) ;
#34566=VERTEX_POINT('',#124550) ;
#34567=VERTEX_POINT('',#124551) ;
#34568=VERTEX_POINT('',#124626) ;
#34569=VERTEX_POINT('',#124627) ;
#34570=VERTEX_POINT('',#124706) ;
#34571=VERTEX_POINT('',#124707) ;
#34572=VERTEX_POINT('',#124782) ;
#34573=VERTEX_POINT('',#124783) ;
#34574=VERTEX_POINT('',#124785) ;
#34575=VERTEX_POINT('',#124798) ;
#34576=VERTEX_POINT('',#124809) ;
#34577=VERTEX_POINT('',#124810) ;
#34578=VERTEX_POINT('',#124885) ;
#34579=VERTEX_POINT('',#124886) ;
#34580=VERTEX_POINT('',#124961) ;
#34581=VERTEX_POINT('',#124962) ;
#34582=VERTEX_POINT('',#125037) ;
#34583=VERTEX_POINT('',#125038) ;
#34584=VERTEX_POINT('',#125113) ;
#34585=VERTEX_POINT('',#125114) ;
#34586=VERTEX_POINT('',#125189) ;
#34587=VERTEX_POINT('',#125190) ;
#34588=VERTEX_POINT('',#125267) ;
#34589=VERTEX_POINT('',#125268) ;
#34590=VERTEX_POINT('',#125345) ;
#34591=VERTEX_POINT('',#125347) ;
#34592=VERTEX_POINT('',#125349) ;
#34593=VERTEX_POINT('',#125378) ;
#34594=VERTEX_POINT('',#125380) ;
#34595=VERTEX_POINT('',#125382) ;
#34596=VERTEX_POINT('',#125384) ;
#34597=VERTEX_POINT('',#125415) ;
#34598=VERTEX_POINT('',#125527) ;
#34599=VERTEX_POINT('',#125550) ;
#34600=VERTEX_POINT('',#125567) ;
#34601=VERTEX_POINT('',#125569) ;
#34602=VERTEX_POINT('',#125573) ;
#34603=VERTEX_POINT('',#125577) ;
#34604=VERTEX_POINT('',#125580) ;
#34605=VERTEX_POINT('',#125584) ;
#34606=VERTEX_POINT('',#125615) ;
#34607=VERTEX_POINT('',#125639) ;
#34608=VERTEX_POINT('',#125640) ;
#34609=VERTEX_POINT('',#125642) ;
#34610=VERTEX_POINT('',#125644) ;
#34611=VERTEX_POINT('',#125648) ;
#34612=VERTEX_POINT('',#125649) ;
#34613=VERTEX_POINT('',#125651) ;
#34614=VERTEX_POINT('',#125653) ;
#34615=VERTEX_POINT('',#125657) ;
#34616=VERTEX_POINT('',#125658) ;
#34617=VERTEX_POINT('',#125660) ;
#34618=VERTEX_POINT('',#125662) ;
#34619=VERTEX_POINT('',#125666) ;
#34620=VERTEX_POINT('',#125667) ;
#34621=VERTEX_POINT('',#125669) ;
#34622=VERTEX_POINT('',#125671) ;
#34623=VERTEX_POINT('',#125675) ;
#34624=VERTEX_POINT('',#125676) ;
#34625=VERTEX_POINT('',#125678) ;
#34626=VERTEX_POINT('',#125680) ;
#34627=VERTEX_POINT('',#125684) ;
#34628=VERTEX_POINT('',#125685) ;
#34629=VERTEX_POINT('',#125687) ;
#34630=VERTEX_POINT('',#125689) ;
#34631=VERTEX_POINT('',#125693) ;
#34632=VERTEX_POINT('',#125697) ;
#34633=VERTEX_POINT('',#125703) ;
#34634=VERTEX_POINT('',#125712) ;
#34635=VERTEX_POINT('',#125721) ;
#34636=VERTEX_POINT('',#125730) ;
#34637=VERTEX_POINT('',#125747) ;
#34638=VERTEX_POINT('',#125751) ;
#34639=VERTEX_POINT('',#125757) ;
#34640=VERTEX_POINT('',#125769) ;
#34641=VERTEX_POINT('',#125778) ;
#34642=VERTEX_POINT('',#125787) ;
#34643=VERTEX_POINT('',#126350) ;
#43838=EDGE_CURVE('',#34550,#34551,#11944,.T.) ;
#43839=EDGE_CURVE('',#34550,#34552,#330,.T.) ;
#43840=EDGE_CURVE('',#34552,#34553,#11945,.T.) ;
#43841=EDGE_CURVE('',#34551,#34553,#331,.F.) ;
#43842=EDGE_CURVE('',#34554,#34555,#11946,.T.) ;
#43843=EDGE_CURVE('',#34554,#34550,#332,.T.) ;
#43844=EDGE_CURVE('',#34555,#34551,#333,.F.) ;
#43845=EDGE_CURVE('',#34556,#34557,#11947,.T.) ;
#43846=EDGE_CURVE('',#34556,#34554,#334,.T.) ;
#43847=EDGE_CURVE('',#34557,#34555,#335,.F.) ;
#43848=EDGE_CURVE('',#34558,#34559,#11948,.T.) ;
#43849=EDGE_CURVE('',#34558,#34556,#336,.T.) ;
#43850=EDGE_CURVE('',#34559,#34557,#337,.F.) ;
#43851=EDGE_CURVE('',#34560,#34561,#11949,.T.) ;
#43852=EDGE_CURVE('',#34560,#34558,#338,.T.) ;
#43853=EDGE_CURVE('',#34561,#34559,#339,.F.) ;
#43854=EDGE_CURVE('',#34562,#34563,#11950,.T.) ;
#43855=EDGE_CURVE('',#34562,#34560,#340,.T.) ;
#43856=EDGE_CURVE('',#34563,#34561,#341,.F.) ;
#43857=EDGE_CURVE('',#34564,#34565,#11951,.T.) ;
#43858=EDGE_CURVE('',#34564,#34562,#342,.T.) ;
#43859=EDGE_CURVE('',#34565,#34563,#343,.F.) ;
#43860=EDGE_CURVE('',#34566,#34567,#11952,.T.) ;
#43861=EDGE_CURVE('',#34566,#34564,#344,.T.) ;
#43862=EDGE_CURVE('',#34567,#34565,#345,.F.) ;
#43863=EDGE_CURVE('',#34568,#34569,#11953,.T.) ;
#43864=EDGE_CURVE('',#34568,#34566,#346,.T.) ;
#43865=EDGE_CURVE('',#34569,#34567,#347,.F.) ;
#43866=EDGE_CURVE('',#34570,#34571,#11954,.T.) ;
#43867=EDGE_CURVE('',#34570,#34568,#348,.T.) ;
#43868=EDGE_CURVE('',#34571,#34569,#349,.F.) ;
#43869=EDGE_CURVE('',#34572,#34573,#11955,.T.) ;
#43870=EDGE_CURVE('',#34574,#34572,#350,.F.) ;
#43871=EDGE_CURVE('',#34574,#34575,#29419,.T.) ;
#43872=EDGE_CURVE('',#34575,#34573,#351,.T.) ;
#43873=EDGE_CURVE('',#34576,#34577,#11956,.T.) ;
#43874=EDGE_CURVE('',#34572,#34576,#352,.F.) ;
#43875=EDGE_CURVE('',#34573,#34577,#353,.T.) ;
#43876=EDGE_CURVE('',#34578,#34579,#11957,.T.) ;
#43877=EDGE_CURVE('',#34576,#34578,#354,.F.) ;
#43878=EDGE_CURVE('',#34577,#34579,#355,.T.) ;
#43879=EDGE_CURVE('',#34580,#34581,#11958,.T.) ;
#43880=EDGE_CURVE('',#34578,#34580,#356,.F.) ;
#43881=EDGE_CURVE('',#34579,#34581,#357,.T.) ;
#43882=EDGE_CURVE('',#34582,#34583,#11959,.T.) ;
#43883=EDGE_CURVE('',#34580,#34582,#358,.F.) ;
#43884=EDGE_CURVE('',#34581,#34583,#359,.T.) ;
#43885=EDGE_CURVE('',#34584,#34585,#11960,.T.) ;
#43886=EDGE_CURVE('',#34582,#34584,#360,.F.) ;
#43887=EDGE_CURVE('',#34583,#34585,#361,.T.) ;
#43888=EDGE_CURVE('',#34586,#34587,#11961,.T.) ;
#43889=EDGE_CURVE('',#34584,#34586,#362,.F.) ;
#43890=EDGE_CURVE('',#34585,#34587,#363,.T.) ;
#43891=EDGE_CURVE('',#34588,#34589,#11962,.T.) ;
#43892=EDGE_CURVE('',#34586,#34588,#364,.F.) ;
#43893=EDGE_CURVE('',#34587,#34589,#365,.T.) ;
#43894=EDGE_CURVE('',#34590,#34590,#29420,.T.) ;
#43895=EDGE_CURVE('',#34590,#34591,#11963,.T.) ;
#43896=EDGE_CURVE('',#34591,#34592,#366,.T.) ;
#43897=EDGE_CURVE('',#34592,#34593,#4983,.T.) ;
#43898=EDGE_CURVE('',#34593,#34594,#11964,.T.) ;
#43899=EDGE_CURVE('',#34594,#34595,#4984,.T.) ;
#43900=EDGE_CURVE('',#34596,#34595,#367,.F.) ;
#43901=EDGE_CURVE('',#34596,#34597,#11965,.T.) ;
#43902=EDGE_CURVE('',#34597,#34591,#368,.T.) ;
#43903=EDGE_CURVE('',#34588,#34596,#369,.F.) ;
#43904=EDGE_CURVE('',#34589,#34597,#370,.T.) ;
#43905=EDGE_CURVE('',#34598,#34571,#371,.F.) ;
#43906=EDGE_CURVE('',#34599,#34598,#29421,.T.) ;
#43907=EDGE_CURVE('',#34599,#34570,#372,.T.) ;
#43908=EDGE_CURVE('',#34600,#34600,#29422,.T.) ;
#43909=EDGE_CURVE('',#34600,#34601,#11966,.T.) ;
#43910=EDGE_CURVE('',#34601,#34601,#29423,.T.) ;
#43911=EDGE_CURVE('',#34602,#34602,#29424,.T.) ;
#43912=EDGE_CURVE('',#34602,#34600,#11967,.T.) ;
#43913=EDGE_CURVE('',#34603,#34602,#11968,.T.) ;
#43914=EDGE_CURVE('',#34604,#34604,#29425,.T.) ;
#43915=EDGE_CURVE('',#34604,#34590,#29426,.T.) ;
#43916=EDGE_CURVE('',#34574,#34605,#373,.F.) ;
#43917=EDGE_CURVE('',#34605,#34606,#11969,.T.) ;
#43918=EDGE_CURVE('',#34606,#34606,#29427,.T.) ;
#43919=EDGE_CURVE('',#34605,#34599,#374,.F.) ;
#43920=EDGE_CURVE('',#34598,#34575,#375,.T.) ;
#43921=EDGE_CURVE('',#34607,#34608,#11970,.T.) ;
#43922=EDGE_CURVE('',#34607,#34609,#29428,.T.) ;
#43923=EDGE_CURVE('',#34610,#34609,#11971,.T.) ;
#43924=EDGE_CURVE('',#34610,#34608,#29429,.T.) ;
#43925=EDGE_CURVE('',#34611,#34612,#11972,.T.) ;
#43926=EDGE_CURVE('',#34611,#34613,#29430,.T.) ;
#43927=EDGE_CURVE('',#34614,#34613,#11973,.T.) ;
#43928=EDGE_CURVE('',#34614,#34612,#29431,.T.) ;
#43929=EDGE_CURVE('',#34615,#34616,#11974,.T.) ;
#43930=EDGE_CURVE('',#34615,#34617,#29432,.T.) ;
#43931=EDGE_CURVE('',#34618,#34617,#11975,.T.) ;
#43932=EDGE_CURVE('',#34618,#34616,#29433,.T.) ;
#43933=EDGE_CURVE('',#34619,#34620,#11976,.T.) ;
#43934=EDGE_CURVE('',#34619,#34621,#29434,.T.) ;
#43935=EDGE_CURVE('',#34622,#34621,#11977,.T.) ;
#43936=EDGE_CURVE('',#34622,#34620,#29435,.T.) ;
#43937=EDGE_CURVE('',#34623,#34624,#11978,.T.) ;
#43938=EDGE_CURVE('',#34623,#34625,#29436,.T.) ;
#43939=EDGE_CURVE('',#34626,#34625,#11979,.T.) ;
#43940=EDGE_CURVE('',#34626,#34624,#29437,.T.) ;
#43941=EDGE_CURVE('',#34627,#34628,#11980,.T.) ;
#43942=EDGE_CURVE('',#34627,#34629,#29438,.T.) ;
#43943=EDGE_CURVE('',#34630,#34629,#11981,.T.) ;
#43944=EDGE_CURVE('',#34630,#34628,#29439,.T.) ;
#43945=EDGE_CURVE('',#34611,#34631,#43,.T.) ;
#43946=EDGE_CURVE('',#34632,#34631,#29440,.T.) ;
#43947=EDGE_CURVE('',#34632,#34613,#44,.T.) ;
#43948=EDGE_CURVE('',#34631,#34633,#29441,.T.) ;
#43949=EDGE_CURVE('',#34631,#34608,#45,.T.) ;
#43950=EDGE_CURVE('',#34610,#34633,#46,.T.) ;
#43951=EDGE_CURVE('',#34633,#34634,#29442,.T.) ;
#43952=EDGE_CURVE('',#34633,#34616,#47,.T.) ;
#43953=EDGE_CURVE('',#34618,#34634,#48,.T.) ;
#43954=EDGE_CURVE('',#34634,#34635,#29443,.T.) ;
#43955=EDGE_CURVE('',#34634,#34620,#49,.T.) ;
#43956=EDGE_CURVE('',#34622,#34635,#50,.T.) ;
#43957=EDGE_CURVE('',#34635,#34636,#29444,.T.) ;
#43958=EDGE_CURVE('',#34635,#34624,#51,.T.) ;
#43959=EDGE_CURVE('',#34626,#34636,#52,.T.) ;
#43960=EDGE_CURVE('',#34636,#34632,#29445,.T.) ;
#43961=EDGE_CURVE('',#34636,#34628,#53,.T.) ;
#43962=EDGE_CURVE('',#34630,#34632,#54,.T.) ;
#43963=EDGE_CURVE('',#34607,#34637,#55,.T.) ;
#43964=EDGE_CURVE('',#34638,#34637,#29446,.T.) ;
#43965=EDGE_CURVE('',#34638,#34609,#56,.T.) ;
#43966=EDGE_CURVE('',#34637,#34639,#29447,.T.) ;
#43967=EDGE_CURVE('',#34637,#34612,#57,.T.) ;
#43968=EDGE_CURVE('',#34614,#34639,#58,.T.) ;
#43969=EDGE_CURVE('',#34615,#34638,#59,.T.) ;
#43970=EDGE_CURVE('',#34640,#34638,#29448,.T.) ;
#43971=EDGE_CURVE('',#34640,#34617,#60,.T.) ;
#43972=EDGE_CURVE('',#34619,#34640,#61,.T.) ;
#43973=EDGE_CURVE('',#34641,#34640,#29449,.T.) ;
#43974=EDGE_CURVE('',#34641,#34621,#62,.T.) ;
#43975=EDGE_CURVE('',#34623,#34641,#63,.T.) ;
#43976=EDGE_CURVE('',#34642,#34641,#29450,.T.) ;
#43977=EDGE_CURVE('',#34642,#34625,#64,.T.) ;
#43978=EDGE_CURVE('',#34627,#34642,#65,.T.) ;
#43979=EDGE_CURVE('',#34639,#34642,#29451,.T.) ;
#43980=EDGE_CURVE('',#34639,#34629,#66,.T.) ;
#43981=EDGE_CURVE('',#34595,#34552,#11982,.T.) ;
#43982=EDGE_CURVE('',#34643,#34553,#29452,.T.) ;
#43983=EDGE_CURVE('',#34592,#34643,#376,.T.) ;
#43984=EDGE_CURVE('',#34594,#34552,#11983,.T.) ;
#43985=EDGE_CURVE('',#34593,#34553,#11984,.T.) ;
#62358=ORIENTED_EDGE('',*,*,#43838,.F.) ;
#62359=ORIENTED_EDGE('',*,*,#43839,.T.) ;
#62360=ORIENTED_EDGE('',*,*,#43840,.T.) ;
#62361=ORIENTED_EDGE('',*,*,#43841,.F.) ;
#62362=ORIENTED_EDGE('',*,*,#43842,.F.) ;
#62363=ORIENTED_EDGE('',*,*,#43843,.T.) ;
#62364=ORIENTED_EDGE('',*,*,#43838,.T.) ;
#62365=ORIENTED_EDGE('',*,*,#43844,.F.) ;
#62366=ORIENTED_EDGE('',*,*,#43845,.F.) ;
#62367=ORIENTED_EDGE('',*,*,#43846,.T.) ;
#62368=ORIENTED_EDGE('',*,*,#43842,.T.) ;
#62369=ORIENTED_EDGE('',*,*,#43847,.F.) ;
#62370=ORIENTED_EDGE('',*,*,#43848,.F.) ;
#62371=ORIENTED_EDGE('',*,*,#43849,.T.) ;
#62372=ORIENTED_EDGE('',*,*,#43845,.T.) ;
#62373=ORIENTED_EDGE('',*,*,#43850,.F.) ;
#62374=ORIENTED_EDGE('',*,*,#43851,.F.) ;
#62375=ORIENTED_EDGE('',*,*,#43852,.T.) ;
#62376=ORIENTED_EDGE('',*,*,#43848,.T.) ;
#62377=ORIENTED_EDGE('',*,*,#43853,.F.) ;
#62378=ORIENTED_EDGE('',*,*,#43854,.F.) ;
#62379=ORIENTED_EDGE('',*,*,#43855,.T.) ;
#62380=ORIENTED_EDGE('',*,*,#43851,.T.) ;
#62381=ORIENTED_EDGE('',*,*,#43856,.F.) ;
#62382=ORIENTED_EDGE('',*,*,#43857,.F.) ;
#62383=ORIENTED_EDGE('',*,*,#43858,.T.) ;
#62384=ORIENTED_EDGE('',*,*,#43854,.T.) ;
#62385=ORIENTED_EDGE('',*,*,#43859,.F.) ;
#62386=ORIENTED_EDGE('',*,*,#43860,.F.) ;
#62387=ORIENTED_EDGE('',*,*,#43861,.T.) ;
#62388=ORIENTED_EDGE('',*,*,#43857,.T.) ;
#62389=ORIENTED_EDGE('',*,*,#43862,.F.) ;
#62390=ORIENTED_EDGE('',*,*,#43863,.F.) ;
#62391=ORIENTED_EDGE('',*,*,#43864,.T.) ;
#62392=ORIENTED_EDGE('',*,*,#43860,.T.) ;
#62393=ORIENTED_EDGE('',*,*,#43865,.F.) ;
#62394=ORIENTED_EDGE('',*,*,#43866,.F.) ;
#62395=ORIENTED_EDGE('',*,*,#43867,.T.) ;
#62396=ORIENTED_EDGE('',*,*,#43863,.T.) ;
#62397=ORIENTED_EDGE('',*,*,#43868,.F.) ;
#62398=ORIENTED_EDGE('',*,*,#43869,.F.) ;
#62399=ORIENTED_EDGE('',*,*,#43870,.F.) ;
#62400=ORIENTED_EDGE('',*,*,#43871,.T.) ;
#62401=ORIENTED_EDGE('',*,*,#43872,.T.) ;
#62402=ORIENTED_EDGE('',*,*,#43873,.F.) ;
#62403=ORIENTED_EDGE('',*,*,#43874,.F.) ;
#62404=ORIENTED_EDGE('',*,*,#43869,.T.) ;
#62405=ORIENTED_EDGE('',*,*,#43875,.T.) ;
#62406=ORIENTED_EDGE('',*,*,#43876,.F.) ;
#62407=ORIENTED_EDGE('',*,*,#43877,.F.) ;
#62408=ORIENTED_EDGE('',*,*,#43873,.T.) ;
#62409=ORIENTED_EDGE('',*,*,#43878,.T.) ;
#62410=ORIENTED_EDGE('',*,*,#43879,.F.) ;
#62411=ORIENTED_EDGE('',*,*,#43880,.F.) ;
#62412=ORIENTED_EDGE('',*,*,#43876,.T.) ;
#62413=ORIENTED_EDGE('',*,*,#43881,.T.) ;
#62414=ORIENTED_EDGE('',*,*,#43882,.F.) ;
#62415=ORIENTED_EDGE('',*,*,#43883,.F.) ;
#62416=ORIENTED_EDGE('',*,*,#43879,.T.) ;
#62417=ORIENTED_EDGE('',*,*,#43884,.T.) ;
#62418=ORIENTED_EDGE('',*,*,#43885,.F.) ;
#62419=ORIENTED_EDGE('',*,*,#43886,.F.) ;
#62420=ORIENTED_EDGE('',*,*,#43882,.T.) ;
#62421=ORIENTED_EDGE('',*,*,#43887,.T.) ;
#62422=ORIENTED_EDGE('',*,*,#43888,.F.) ;
#62423=ORIENTED_EDGE('',*,*,#43889,.F.) ;
#62424=ORIENTED_EDGE('',*,*,#43885,.T.) ;
#62425=ORIENTED_EDGE('',*,*,#43890,.T.) ;
#62426=ORIENTED_EDGE('',*,*,#43891,.F.) ;
#62427=ORIENTED_EDGE('',*,*,#43892,.F.) ;
#62428=ORIENTED_EDGE('',*,*,#43888,.T.) ;
#62429=ORIENTED_EDGE('',*,*,#43893,.T.) ;
#62430=ORIENTED_EDGE('',*,*,#43894,.T.) ;
#62431=ORIENTED_EDGE('',*,*,#43895,.T.) ;
#62432=ORIENTED_EDGE('',*,*,#43896,.T.) ;
#62433=ORIENTED_EDGE('',*,*,#43897,.T.) ;
#62434=ORIENTED_EDGE('',*,*,#43898,.T.) ;
#62435=ORIENTED_EDGE('',*,*,#43899,.T.) ;
#62436=ORIENTED_EDGE('',*,*,#43900,.F.) ;
#62437=ORIENTED_EDGE('',*,*,#43901,.T.) ;
#62438=ORIENTED_EDGE('',*,*,#43902,.T.) ;
#62439=ORIENTED_EDGE('',*,*,#43895,.F.) ;
#62440=ORIENTED_EDGE('',*,*,#43901,.F.) ;
#62441=ORIENTED_EDGE('',*,*,#43903,.F.) ;
#62442=ORIENTED_EDGE('',*,*,#43891,.T.) ;
#62443=ORIENTED_EDGE('',*,*,#43904,.T.) ;
#62444=ORIENTED_EDGE('',*,*,#43866,.T.) ;
#62445=ORIENTED_EDGE('',*,*,#43905,.F.) ;
#62446=ORIENTED_EDGE('',*,*,#43906,.F.) ;
#62447=ORIENTED_EDGE('',*,*,#43907,.T.) ;
#62448=ORIENTED_EDGE('',*,*,#43908,.F.) ;
#62449=ORIENTED_EDGE('',*,*,#43909,.T.) ;
#62450=ORIENTED_EDGE('',*,*,#43910,.T.) ;
#62451=ORIENTED_EDGE('',*,*,#43909,.F.) ;
#62452=ORIENTED_EDGE('',*,*,#43911,.F.) ;
#62453=ORIENTED_EDGE('',*,*,#43912,.T.) ;
#62454=ORIENTED_EDGE('',*,*,#43908,.T.) ;
#62455=ORIENTED_EDGE('',*,*,#43912,.F.) ;
#62456=ORIENTED_EDGE('',*,*,#43913,.T.) ;
#62457=ORIENTED_EDGE('',*,*,#43911,.T.) ;
#62458=ORIENTED_EDGE('',*,*,#43913,.F.) ;
#62459=ORIENTED_EDGE('',*,*,#43914,.F.) ;
#62460=ORIENTED_EDGE('',*,*,#43915,.T.) ;
#62461=ORIENTED_EDGE('',*,*,#43894,.F.) ;
#62462=ORIENTED_EDGE('',*,*,#43915,.F.) ;
#62463=ORIENTED_EDGE('',*,*,#43916,.T.) ;
#62464=ORIENTED_EDGE('',*,*,#43917,.T.) ;
#62465=ORIENTED_EDGE('',*,*,#43918,.F.) ;
#62466=ORIENTED_EDGE('',*,*,#43917,.F.) ;
#62467=ORIENTED_EDGE('',*,*,#43919,.T.) ;
#62468=ORIENTED_EDGE('',*,*,#43906,.T.) ;
#62469=ORIENTED_EDGE('',*,*,#43920,.T.) ;
#62470=ORIENTED_EDGE('',*,*,#43871,.F.) ;
#62471=ORIENTED_EDGE('',*,*,#43921,.F.) ;
#62472=ORIENTED_EDGE('',*,*,#43922,.T.) ;
#62473=ORIENTED_EDGE('',*,*,#43923,.F.) ;
#62474=ORIENTED_EDGE('',*,*,#43924,.T.) ;
#62475=ORIENTED_EDGE('',*,*,#43925,.F.) ;
#62476=ORIENTED_EDGE('',*,*,#43926,.T.) ;
#62477=ORIENTED_EDGE('',*,*,#43927,.F.) ;
#62478=ORIENTED_EDGE('',*,*,#43928,.T.) ;
#62479=ORIENTED_EDGE('',*,*,#43929,.F.) ;
#62480=ORIENTED_EDGE('',*,*,#43930,.T.) ;
#62481=ORIENTED_EDGE('',*,*,#43931,.F.) ;
#62482=ORIENTED_EDGE('',*,*,#43932,.T.) ;
#62483=ORIENTED_EDGE('',*,*,#43933,.F.) ;
#62484=ORIENTED_EDGE('',*,*,#43934,.T.) ;
#62485=ORIENTED_EDGE('',*,*,#43935,.F.) ;
#62486=ORIENTED_EDGE('',*,*,#43936,.T.) ;
#62487=ORIENTED_EDGE('',*,*,#43937,.F.) ;
#62488=ORIENTED_EDGE('',*,*,#43938,.T.) ;
#62489=ORIENTED_EDGE('',*,*,#43939,.F.) ;
#62490=ORIENTED_EDGE('',*,*,#43940,.T.) ;
#62491=ORIENTED_EDGE('',*,*,#43941,.F.) ;
#62492=ORIENTED_EDGE('',*,*,#43942,.T.) ;
#62493=ORIENTED_EDGE('',*,*,#43943,.F.) ;
#62494=ORIENTED_EDGE('',*,*,#43944,.T.) ;
#62495=ORIENTED_EDGE('',*,*,#43926,.F.) ;
#62496=ORIENTED_EDGE('',*,*,#43945,.T.) ;
#62497=ORIENTED_EDGE('',*,*,#43946,.F.) ;
#62498=ORIENTED_EDGE('',*,*,#43947,.T.) ;
#62499=ORIENTED_EDGE('',*,*,#43948,.F.) ;
#62500=ORIENTED_EDGE('',*,*,#43949,.T.) ;
#62501=ORIENTED_EDGE('',*,*,#43924,.F.) ;
#62502=ORIENTED_EDGE('',*,*,#43950,.T.) ;
#62503=ORIENTED_EDGE('',*,*,#43951,.F.) ;
#62504=ORIENTED_EDGE('',*,*,#43952,.T.) ;
#62505=ORIENTED_EDGE('',*,*,#43932,.F.) ;
#62506=ORIENTED_EDGE('',*,*,#43953,.T.) ;
#62507=ORIENTED_EDGE('',*,*,#43954,.F.) ;
#62508=ORIENTED_EDGE('',*,*,#43955,.T.) ;
#62509=ORIENTED_EDGE('',*,*,#43936,.F.) ;
#62510=ORIENTED_EDGE('',*,*,#43956,.T.) ;
#62511=ORIENTED_EDGE('',*,*,#43957,.F.) ;
#62512=ORIENTED_EDGE('',*,*,#43958,.T.) ;
#62513=ORIENTED_EDGE('',*,*,#43940,.F.) ;
#62514=ORIENTED_EDGE('',*,*,#43959,.T.) ;
#62515=ORIENTED_EDGE('',*,*,#43960,.F.) ;
#62516=ORIENTED_EDGE('',*,*,#43961,.T.) ;
#62517=ORIENTED_EDGE('',*,*,#43944,.F.) ;
#62518=ORIENTED_EDGE('',*,*,#43962,.T.) ;
#62519=ORIENTED_EDGE('',*,*,#43922,.F.) ;
#62520=ORIENTED_EDGE('',*,*,#43963,.T.) ;
#62521=ORIENTED_EDGE('',*,*,#43964,.F.) ;
#62522=ORIENTED_EDGE('',*,*,#43965,.T.) ;
#62523=ORIENTED_EDGE('',*,*,#43966,.F.) ;
#62524=ORIENTED_EDGE('',*,*,#43967,.T.) ;
#62525=ORIENTED_EDGE('',*,*,#43928,.F.) ;
#62526=ORIENTED_EDGE('',*,*,#43968,.T.) ;
#62527=ORIENTED_EDGE('',*,*,#43930,.F.) ;
#62528=ORIENTED_EDGE('',*,*,#43969,.T.) ;
#62529=ORIENTED_EDGE('',*,*,#43970,.F.) ;
#62530=ORIENTED_EDGE('',*,*,#43971,.T.) ;
#62531=ORIENTED_EDGE('',*,*,#43934,.F.) ;
#62532=ORIENTED_EDGE('',*,*,#43972,.T.) ;
#62533=ORIENTED_EDGE('',*,*,#43973,.F.) ;
#62534=ORIENTED_EDGE('',*,*,#43974,.T.) ;
#62535=ORIENTED_EDGE('',*,*,#43938,.F.) ;
#62536=ORIENTED_EDGE('',*,*,#43975,.T.) ;
#62537=ORIENTED_EDGE('',*,*,#43976,.F.) ;
#62538=ORIENTED_EDGE('',*,*,#43977,.T.) ;
#62539=ORIENTED_EDGE('',*,*,#43942,.F.) ;
#62540=ORIENTED_EDGE('',*,*,#43978,.T.) ;
#62541=ORIENTED_EDGE('',*,*,#43979,.F.) ;
#62542=ORIENTED_EDGE('',*,*,#43980,.T.) ;
#62543=ORIENTED_EDGE('',*,*,#43964,.T.) ;
#62544=ORIENTED_EDGE('',*,*,#43966,.T.) ;
#62545=ORIENTED_EDGE('',*,*,#43979,.T.) ;
#62546=ORIENTED_EDGE('',*,*,#43976,.T.) ;
#62547=ORIENTED_EDGE('',*,*,#43973,.T.) ;
#62548=ORIENTED_EDGE('',*,*,#43970,.T.) ;
#62549=ORIENTED_EDGE('',*,*,#43910,.F.) ;
#62550=ORIENTED_EDGE('',*,*,#43951,.T.) ;
#62551=ORIENTED_EDGE('',*,*,#43954,.T.) ;
#62552=ORIENTED_EDGE('',*,*,#43957,.T.) ;
#62553=ORIENTED_EDGE('',*,*,#43960,.T.) ;
#62554=ORIENTED_EDGE('',*,*,#43946,.T.) ;
#62555=ORIENTED_EDGE('',*,*,#43948,.T.) ;
#62556=ORIENTED_EDGE('',*,*,#43914,.T.) ;
#62557=ORIENTED_EDGE('',*,*,#43918,.T.) ;
#62558=ORIENTED_EDGE('',*,*,#43943,.T.) ;
#62559=ORIENTED_EDGE('',*,*,#43980,.F.) ;
#62560=ORIENTED_EDGE('',*,*,#43968,.F.) ;
#62561=ORIENTED_EDGE('',*,*,#43927,.T.) ;
#62562=ORIENTED_EDGE('',*,*,#43947,.F.) ;
#62563=ORIENTED_EDGE('',*,*,#43962,.F.) ;
#62564=ORIENTED_EDGE('',*,*,#43939,.T.) ;
#62565=ORIENTED_EDGE('',*,*,#43977,.F.) ;
#62566=ORIENTED_EDGE('',*,*,#43978,.F.) ;
#62567=ORIENTED_EDGE('',*,*,#43941,.T.) ;
#62568=ORIENTED_EDGE('',*,*,#43961,.F.) ;
#62569=ORIENTED_EDGE('',*,*,#43959,.F.) ;
#62570=ORIENTED_EDGE('',*,*,#43935,.T.) ;
#62571=ORIENTED_EDGE('',*,*,#43974,.F.) ;
#62572=ORIENTED_EDGE('',*,*,#43975,.F.) ;
#62573=ORIENTED_EDGE('',*,*,#43937,.T.) ;
#62574=ORIENTED_EDGE('',*,*,#43958,.F.) ;
#62575=ORIENTED_EDGE('',*,*,#43956,.F.) ;
#62576=ORIENTED_EDGE('',*,*,#43931,.T.) ;
#62577=ORIENTED_EDGE('',*,*,#43971,.F.) ;
#62578=ORIENTED_EDGE('',*,*,#43972,.F.) ;
#62579=ORIENTED_EDGE('',*,*,#43933,.T.) ;
#62580=ORIENTED_EDGE('',*,*,#43955,.F.) ;
#62581=ORIENTED_EDGE('',*,*,#43953,.F.) ;
#62582=ORIENTED_EDGE('',*,*,#43923,.T.) ;
#62583=ORIENTED_EDGE('',*,*,#43965,.F.) ;
#62584=ORIENTED_EDGE('',*,*,#43969,.F.) ;
#62585=ORIENTED_EDGE('',*,*,#43929,.T.) ;
#62586=ORIENTED_EDGE('',*,*,#43952,.F.) ;
#62587=ORIENTED_EDGE('',*,*,#43950,.F.) ;
#62588=ORIENTED_EDGE('',*,*,#43925,.T.) ;
#62589=ORIENTED_EDGE('',*,*,#43967,.F.) ;
#62590=ORIENTED_EDGE('',*,*,#43963,.F.) ;
#62591=ORIENTED_EDGE('',*,*,#43921,.T.) ;
#62592=ORIENTED_EDGE('',*,*,#43949,.F.) ;
#62593=ORIENTED_EDGE('',*,*,#43945,.F.) ;
#62594=ORIENTED_EDGE('',*,*,#43870,.T.) ;
#62595=ORIENTED_EDGE('',*,*,#43874,.T.) ;
#62596=ORIENTED_EDGE('',*,*,#43877,.T.) ;
#62597=ORIENTED_EDGE('',*,*,#43880,.T.) ;
#62598=ORIENTED_EDGE('',*,*,#43883,.T.) ;
#62599=ORIENTED_EDGE('',*,*,#43886,.T.) ;
#62600=ORIENTED_EDGE('',*,*,#43889,.T.) ;
#62601=ORIENTED_EDGE('',*,*,#43892,.T.) ;
#62602=ORIENTED_EDGE('',*,*,#43903,.T.) ;
#62603=ORIENTED_EDGE('',*,*,#43900,.T.) ;
#62604=ORIENTED_EDGE('',*,*,#43981,.T.) ;
#62605=ORIENTED_EDGE('',*,*,#43839,.F.) ;
#62606=ORIENTED_EDGE('',*,*,#43843,.F.) ;
#62607=ORIENTED_EDGE('',*,*,#43846,.F.) ;
#62608=ORIENTED_EDGE('',*,*,#43849,.F.) ;
#62609=ORIENTED_EDGE('',*,*,#43852,.F.) ;
#62610=ORIENTED_EDGE('',*,*,#43855,.F.) ;
#62611=ORIENTED_EDGE('',*,*,#43858,.F.) ;
#62612=ORIENTED_EDGE('',*,*,#43861,.F.) ;
#62613=ORIENTED_EDGE('',*,*,#43864,.F.) ;
#62614=ORIENTED_EDGE('',*,*,#43867,.F.) ;
#62615=ORIENTED_EDGE('',*,*,#43907,.F.) ;
#62616=ORIENTED_EDGE('',*,*,#43919,.F.) ;
#62617=ORIENTED_EDGE('',*,*,#43916,.F.) ;
#62618=ORIENTED_EDGE('',*,*,#43982,.F.) ;
#62619=ORIENTED_EDGE('',*,*,#43983,.F.) ;
#62620=ORIENTED_EDGE('',*,*,#43896,.F.) ;
#62621=ORIENTED_EDGE('',*,*,#43902,.F.) ;
#62622=ORIENTED_EDGE('',*,*,#43904,.F.) ;
#62623=ORIENTED_EDGE('',*,*,#43893,.F.) ;
#62624=ORIENTED_EDGE('',*,*,#43890,.F.) ;
#62625=ORIENTED_EDGE('',*,*,#43887,.F.) ;
#62626=ORIENTED_EDGE('',*,*,#43884,.F.) ;
#62627=ORIENTED_EDGE('',*,*,#43881,.F.) ;
#62628=ORIENTED_EDGE('',*,*,#43878,.F.) ;
#62629=ORIENTED_EDGE('',*,*,#43875,.F.) ;
#62630=ORIENTED_EDGE('',*,*,#43872,.F.) ;
#62631=ORIENTED_EDGE('',*,*,#43920,.F.) ;
#62632=ORIENTED_EDGE('',*,*,#43905,.T.) ;
#62633=ORIENTED_EDGE('',*,*,#43868,.T.) ;
#62634=ORIENTED_EDGE('',*,*,#43865,.T.) ;
#62635=ORIENTED_EDGE('',*,*,#43862,.T.) ;
#62636=ORIENTED_EDGE('',*,*,#43859,.T.) ;
#62637=ORIENTED_EDGE('',*,*,#43856,.T.) ;
#62638=ORIENTED_EDGE('',*,*,#43853,.T.) ;
#62639=ORIENTED_EDGE('',*,*,#43850,.T.) ;
#62640=ORIENTED_EDGE('',*,*,#43847,.T.) ;
#62641=ORIENTED_EDGE('',*,*,#43844,.T.) ;
#62642=ORIENTED_EDGE('',*,*,#43841,.T.) ;
#62643=ORIENTED_EDGE('',*,*,#43984,.T.) ;
#62644=ORIENTED_EDGE('',*,*,#43981,.F.) ;
#62645=ORIENTED_EDGE('',*,*,#43899,.F.) ;
#62646=ORIENTED_EDGE('',*,*,#43985,.T.) ;
#62647=ORIENTED_EDGE('',*,*,#43840,.F.) ;
#62648=ORIENTED_EDGE('',*,*,#43984,.F.) ;
#62649=ORIENTED_EDGE('',*,*,#43898,.F.) ;
#62650=ORIENTED_EDGE('',*,*,#43983,.T.) ;
#62651=ORIENTED_EDGE('',*,*,#43982,.T.) ;
#62652=ORIENTED_EDGE('',*,*,#43985,.F.) ;
#62653=ORIENTED_EDGE('',*,*,#43897,.F.) ;
#63441=TOROIDAL_SURFACE('',#76702,1.6,0.1) ;
#67592=ADVANCED_FACE('',(#20307),#7866,.T.) ;
#67593=ADVANCED_FACE('',(#20308),#7867,.T.) ;
#67594=ADVANCED_FACE('',(#20309),#7868,.T.) ;
#67595=ADVANCED_FACE('',(#20310),#7869,.T.) ;
#67596=ADVANCED_FACE('',(#20311),#7870,.T.) ;
#67597=ADVANCED_FACE('',(#20312),#7871,.T.) ;
#67598=ADVANCED_FACE('',(#20313),#7872,.T.) ;
#67599=ADVANCED_FACE('',(#20314),#7873,.T.) ;
#67600=ADVANCED_FACE('',(#20315),#7874,.T.) ;
#67601=ADVANCED_FACE('',(#20316),#7875,.T.) ;
#67602=ADVANCED_FACE('',(#20317),#7876,.T.) ;
#67603=ADVANCED_FACE('',(#20318),#7877,.T.) ;
#67604=ADVANCED_FACE('',(#20319),#7878,.T.) ;
#67605=ADVANCED_FACE('',(#20320),#7879,.T.) ;
#67606=ADVANCED_FACE('',(#20321),#7880,.T.) ;
#67607=ADVANCED_FACE('',(#20322),#7881,.T.) ;
#67608=ADVANCED_FACE('',(#20323),#7882,.T.) ;
#67609=ADVANCED_FACE('',(#20324),#7883,.T.) ;
#67610=ADVANCED_FACE('',(#20325),#7884,.T.) ;
#67611=ADVANCED_FACE('',(#20326),#7885,.T.) ;
#67612=ADVANCED_FACE('',(#20327),#7886,.T.) ;
#67613=ADVANCED_FACE('',(#20328),#16135,.F.) ;
#67614=ADVANCED_FACE('',(#20329),#7887,.F.) ;
#67615=ADVANCED_FACE('',(#20330),#16136,.F.) ;
#67616=ADVANCED_FACE('',(#20331),#63441,.F.) ;
#67617=ADVANCED_FACE('',(#20332),#16137,.T.) ;
#67618=ADVANCED_FACE('',(#20333),#7888,.T.) ;
#67619=ADVANCED_FACE('',(#20334),#7889,.T.) ;
#67620=ADVANCED_FACE('',(#20335),#7890,.T.) ;
#67621=ADVANCED_FACE('',(#20336),#7891,.T.) ;
#67622=ADVANCED_FACE('',(#20337),#7892,.T.) ;
#67623=ADVANCED_FACE('',(#20338),#7893,.T.) ;
#67624=ADVANCED_FACE('',(#20339),#16138,.T.) ;
#67625=ADVANCED_FACE('',(#20340),#16139,.T.) ;
#67626=ADVANCED_FACE('',(#20341),#16140,.T.) ;
#67627=ADVANCED_FACE('',(#20342),#16141,.T.) ;
#67628=ADVANCED_FACE('',(#20343),#16142,.T.) ;
#67629=ADVANCED_FACE('',(#20344),#16143,.T.) ;
#67630=ADVANCED_FACE('',(#20345),#16144,.T.) ;
#67631=ADVANCED_FACE('',(#20346),#16145,.T.) ;
#67632=ADVANCED_FACE('',(#20347),#16146,.T.) ;
#67633=ADVANCED_FACE('',(#20348),#16147,.T.) ;
#67634=ADVANCED_FACE('',(#20349),#16148,.T.) ;
#67635=ADVANCED_FACE('',(#20350),#16149,.T.) ;
#67636=ADVANCED_FACE('',(#20351,#5061),#5913,.T.) ;
#67637=ADVANCED_FACE('',(#20352,#5062),#5914,.F.) ;
#67638=ADVANCED_FACE('',(#20353),#5915,.T.) ;
#67639=ADVANCED_FACE('',(#20354),#5916,.T.) ;
#67640=ADVANCED_FACE('',(#20355),#5917,.T.) ;
#67641=ADVANCED_FACE('',(#20356),#5918,.T.) ;
#67642=ADVANCED_FACE('',(#20357),#5919,.T.) ;
#67643=ADVANCED_FACE('',(#20358),#5920,.T.) ;
#67644=ADVANCED_FACE('',(#20359),#5921,.T.) ;
#67645=ADVANCED_FACE('',(#20360),#467,.T.) ;
#67646=ADVANCED_FACE('',(#20361),#468,.T.) ;
#67647=ADVANCED_FACE('',(#20362),#5922,.F.) ;
#67648=ADVANCED_FACE('',(#20363),#5923,.F.) ;
#67649=ADVANCED_FACE('',(#20364),#5924,.F.) ;
#67694=CLOSED_SHELL('',(#67592,#67593,#67594,#67595,#67596,#67597,#67598,
#67599,#67600,#67601,#67602,#67603,#67604,#67605,#67606,#67607,#67608,#67609,
#67610,#67611,#67612,#67613,#67614,#67615,#67616,#67617,#67618,#67619,#67620,
#67621,#67622,#67623,#67624,#67625,#67626,#67627,#67628,#67629,#67630,#67631,
#67632,#67633,#67634,#67635,#67636,#67637,#67638,#67639,#67640,#67641,#67642,
#67643,#67644,#67645,#67646,#67647,#67648,#67649)) ;
#76669=AXIS2_PLACEMENT_3D('',#124041,#98712,#98713) ;
#76670=AXIS2_PLACEMENT_3D('',#124042,#98714,#98715) ;
#76671=AXIS2_PLACEMENT_3D('',#124089,#98718,#98719) ;
#76672=AXIS2_PLACEMENT_3D('',#124169,#98721,#98722) ;
#76673=AXIS2_PLACEMENT_3D('',#124245,#98724,#98725) ;
#76674=AXIS2_PLACEMENT_3D('',#124321,#98727,#98728) ;
#76675=AXIS2_PLACEMENT_3D('',#124397,#98730,#98731) ;
#76676=AXIS2_PLACEMENT_3D('',#124473,#98733,#98734) ;
#76677=AXIS2_PLACEMENT_3D('',#124549,#98736,#98737) ;
#76678=AXIS2_PLACEMENT_3D('',#124625,#98739,#98740) ;
#76679=AXIS2_PLACEMENT_3D('',#124705,#98742,#98743) ;
#76680=AXIS2_PLACEMENT_3D('',#124781,#98745,#98746) ;
#76681=AXIS2_PLACEMENT_3D('',#124799,#98748,#98749) ;
#76682=AXIS2_PLACEMENT_3D('',#124808,#98750,#98751) ;
#76683=AXIS2_PLACEMENT_3D('',#124884,#98753,#98754) ;
#76684=AXIS2_PLACEMENT_3D('',#124960,#98756,#98757) ;
#76685=AXIS2_PLACEMENT_3D('',#125036,#98759,#98760) ;
#76686=AXIS2_PLACEMENT_3D('',#125112,#98762,#98763) ;
#76687=AXIS2_PLACEMENT_3D('',#125188,#98765,#98766) ;
#76688=AXIS2_PLACEMENT_3D('',#125266,#98768,#98769) ;
#76689=AXIS2_PLACEMENT_3D('',#125344,#98771,#98772) ;
#76690=AXIS2_PLACEMENT_3D('',#125346,#98773,#98774) ;
#76691=AXIS2_PLACEMENT_3D('',#125379,#98776,#98777) ;
#76692=AXIS2_PLACEMENT_3D('',#125383,#98779,#98780) ;
#76693=AXIS2_PLACEMENT_3D('',#125453,#98782,#98783) ;
#76694=AXIS2_PLACEMENT_3D('',#125526,#98784,#98785) ;
#76695=AXIS2_PLACEMENT_3D('',#125551,#98786,#98787) ;
#76696=AXIS2_PLACEMENT_3D('',#125566,#98788,#98789) ;
#76697=AXIS2_PLACEMENT_3D('',#125568,#98790,#98791) ;
#76698=AXIS2_PLACEMENT_3D('',#125571,#98793,#98794) ;
#76699=AXIS2_PLACEMENT_3D('',#125572,#98795,#98796) ;
#76700=AXIS2_PLACEMENT_3D('',#125574,#98797,#98798) ;
#76701=AXIS2_PLACEMENT_3D('',#125576,#98800,#98801) ;
#76702=AXIS2_PLACEMENT_3D('',#125579,#98803,#98804) ;
#76703=AXIS2_PLACEMENT_3D('',#125581,#98805,#98806) ;
#76704=AXIS2_PLACEMENT_3D('',#125582,#98807,#98808) ;
#76705=AXIS2_PLACEMENT_3D('',#125583,#98809,#98810) ;
#76706=AXIS2_PLACEMENT_3D('',#125617,#98812,#98813) ;
#76707=AXIS2_PLACEMENT_3D('',#125638,#98814,#98815) ;
#76708=AXIS2_PLACEMENT_3D('',#125643,#98817,#98818) ;
#76709=AXIS2_PLACEMENT_3D('',#125646,#98820,#98821) ;
#76710=AXIS2_PLACEMENT_3D('',#125647,#98822,#98823) ;
#76711=AXIS2_PLACEMENT_3D('',#125652,#98825,#98826) ;
#76712=AXIS2_PLACEMENT_3D('',#125655,#98828,#98829) ;
#76713=AXIS2_PLACEMENT_3D('',#125656,#98830,#98831) ;
#76714=AXIS2_PLACEMENT_3D('',#125661,#98833,#98834) ;
#76715=AXIS2_PLACEMENT_3D('',#125664,#98836,#98837) ;
#76716=AXIS2_PLACEMENT_3D('',#125665,#98838,#98839) ;
#76717=AXIS2_PLACEMENT_3D('',#125670,#98841,#98842) ;
#76718=AXIS2_PLACEMENT_3D('',#125673,#98844,#98845) ;
#76719=AXIS2_PLACEMENT_3D('',#125674,#98846,#98847) ;
#76720=AXIS2_PLACEMENT_3D('',#125679,#98849,#98850) ;
#76721=AXIS2_PLACEMENT_3D('',#125682,#98852,#98853) ;
#76722=AXIS2_PLACEMENT_3D('',#125683,#98854,#98855) ;
#76723=AXIS2_PLACEMENT_3D('',#125688,#98857,#98858) ;
#76724=AXIS2_PLACEMENT_3D('',#125691,#98860,#98861) ;
#76725=AXIS2_PLACEMENT_3D('',#125692,#98862,#98863) ;
#76726=AXIS2_PLACEMENT_3D('',#125698,#98864,#98865) ;
#76727=AXIS2_PLACEMENT_3D('',#125702,#98866,#98867) ;
#76728=AXIS2_PLACEMENT_3D('',#125704,#98868,#98869) ;
#76729=AXIS2_PLACEMENT_3D('',#125711,#98870,#98871) ;
#76730=AXIS2_PLACEMENT_3D('',#125713,#98872,#98873) ;
#76731=AXIS2_PLACEMENT_3D('',#125720,#98874,#98875) ;
#76732=AXIS2_PLACEMENT_3D('',#125722,#98876,#98877) ;
#76733=AXIS2_PLACEMENT_3D('',#125729,#98878,#98879) ;
#76734=AXIS2_PLACEMENT_3D('',#125731,#98880,#98881) ;
#76735=AXIS2_PLACEMENT_3D('',#125738,#98882,#98883) ;
#76736=AXIS2_PLACEMENT_3D('',#125739,#98884,#98885) ;
#76737=AXIS2_PLACEMENT_3D('',#125746,#98886,#98887) ;
#76738=AXIS2_PLACEMENT_3D('',#125752,#98888,#98889) ;
#76739=AXIS2_PLACEMENT_3D('',#125756,#98890,#98891) ;
#76740=AXIS2_PLACEMENT_3D('',#125758,#98892,#98893) ;
#76741=AXIS2_PLACEMENT_3D('',#125765,#98894,#98895) ;
#76742=AXIS2_PLACEMENT_3D('',#125770,#98896,#98897) ;
#76743=AXIS2_PLACEMENT_3D('',#125774,#98898,#98899) ;
#76744=AXIS2_PLACEMENT_3D('',#125779,#98900,#98901) ;
#76745=AXIS2_PLACEMENT_3D('',#125783,#98902,#98903) ;
#76746=AXIS2_PLACEMENT_3D('',#125788,#98904,#98905) ;
#76747=AXIS2_PLACEMENT_3D('',#125792,#98906,#98907) ;
#76748=AXIS2_PLACEMENT_3D('',#125796,#98908,#98909) ;
#76749=AXIS2_PLACEMENT_3D('',#125800,#98910,#98911) ;
#76750=AXIS2_PLACEMENT_3D('',#125801,#98912,#98913) ;
#76751=AXIS2_PLACEMENT_3D('',#125802,#98914,#98915) ;
#76752=AXIS2_PLACEMENT_3D('',#125803,#98916,#98917) ;
#76753=AXIS2_PLACEMENT_3D('',#125804,#98918,#98919) ;
#76754=AXIS2_PLACEMENT_3D('',#125805,#98920,#98921) ;
#76755=AXIS2_PLACEMENT_3D('',#125806,#98922,#98923) ;
#76756=AXIS2_PLACEMENT_3D('',#125807,#98924,#98925) ;
#76757=AXIS2_PLACEMENT_3D('',#125808,#98926,#98927) ;
#76758=AXIS2_PLACEMENT_3D('',#126351,#98929,#98930) ;
#76759=AXIS2_PLACEMENT_3D('',#126362,#98931,#98932) ;
#76760=AXIS2_PLACEMENT_3D('',#126364,#98934,#98935) ;
#76761=AXIS2_PLACEMENT_3D('',#126366,#98937,#98938) ;
#98712=DIRECTION('axis',(0.,0.,1.)) ;
#98713=DIRECTION('refdir',(1.,0.,0.)) ;
#98714=DIRECTION('center_axis',(0.,-1.,0.)) ;
#98715=DIRECTION('ref_axis',(1.,0.,2.2577126443575E-16)) ;
#98716=DIRECTION('',(0.,1.,0.)) ;
#98717=DIRECTION('',(2.50091441307106E-5,0.999999996725694,7.6962037204612E-5)) ;
#98718=DIRECTION('center_axis',(0.,-1.,0.)) ;
#98719=DIRECTION('ref_axis',(1.,0.,2.2577126443575E-16)) ;
#98720=DIRECTION('',(0.,1.,0.)) ;
#98721=DIRECTION('center_axis',(0.,-1.,0.)) ;
#98722=DIRECTION('ref_axis',(1.,0.,2.2577126443575E-16)) ;
#98723=DIRECTION('',(0.,1.,0.)) ;
#98724=DIRECTION('center_axis',(0.,-1.,0.)) ;
#98725=DIRECTION('ref_axis',(1.,0.,2.2577126443575E-16)) ;
#98726=DIRECTION('',(0.,1.,0.)) ;
#98727=DIRECTION('center_axis',(0.,-1.,0.)) ;
#98728=DIRECTION('ref_axis',(1.,0.,2.2577126443575E-16)) ;
#98729=DIRECTION('',(0.,1.,0.)) ;
#98730=DIRECTION('center_axis',(0.,-1.,0.)) ;
#98731=DIRECTION('ref_axis',(1.,0.,2.2577126443575E-16)) ;
#98732=DIRECTION('',(0.,1.,0.)) ;
#98733=DIRECTION('center_axis',(0.,-1.,0.)) ;
#98734=DIRECTION('ref_axis',(1.,0.,2.2577126443575E-16)) ;
#98735=DIRECTION('',(0.,1.,0.)) ;
#98736=DIRECTION('center_axis',(0.,-1.,0.)) ;
#98737=DIRECTION('ref_axis',(1.,0.,2.2577126443575E-16)) ;
#98738=DIRECTION('',(0.,1.,0.)) ;
#98739=DIRECTION('center_axis',(0.,-1.,0.)) ;
#98740=DIRECTION('ref_axis',(1.,0.,2.2577126443575E-16)) ;
#98741=DIRECTION('',(0.,1.,0.)) ;
#98742=DIRECTION('center_axis',(0.,-1.,0.)) ;
#98743=DIRECTION('ref_axis',(1.,0.,2.2577126443575E-16)) ;
#98744=DIRECTION('',(0.,1.,0.)) ;
#98745=DIRECTION('center_axis',(0.,1.,0.)) ;
#98746=DIRECTION('ref_axis',(0.,0.,1.)) ;
#98747=DIRECTION('',(0.,-1.,0.)) ;
#98748=DIRECTION('center_axis',(0.,1.,0.)) ;
#98749=DIRECTION('ref_axis',(0.,0.,-1.)) ;
#98750=DIRECTION('center_axis',(0.,1.,0.)) ;
#98751=DIRECTION('ref_axis',(0.,0.,1.)) ;
#98752=DIRECTION('',(0.,-1.,0.)) ;
#98753=DIRECTION('center_axis',(0.,1.,0.)) ;
#98754=DIRECTION('ref_axis',(0.,0.,1.)) ;
#98755=DIRECTION('',(0.,-1.,0.)) ;
#98756=DIRECTION('center_axis',(0.,1.,0.)) ;
#98757=DIRECTION('ref_axis',(0.,0.,1.)) ;
#98758=DIRECTION('',(0.,-1.,0.)) ;
#98759=DIRECTION('center_axis',(0.,1.,0.)) ;
#98760=DIRECTION('ref_axis',(0.,0.,1.)) ;
#98761=DIRECTION('',(0.,-1.,0.)) ;
#98762=DIRECTION('center_axis',(0.,1.,0.)) ;
#98763=DIRECTION('ref_axis',(0.,0.,1.)) ;
#98764=DIRECTION('',(0.,-1.,0.)) ;
#98765=DIRECTION('center_axis',(0.,1.,0.)) ;
#98766=DIRECTION('ref_axis',(0.,0.,1.)) ;
#98767=DIRECTION('',(0.,-1.,0.)) ;
#98768=DIRECTION('center_axis',(0.,1.,0.)) ;
#98769=DIRECTION('ref_axis',(0.,0.,1.)) ;
#98770=DIRECTION('',(0.,-1.,0.)) ;
#98771=DIRECTION('center_axis',(0.,1.,0.)) ;
#98772=DIRECTION('ref_axis',(0.,0.,1.)) ;
#98773=DIRECTION('center_axis',(0.,-1.,0.)) ;
#98774=DIRECTION('ref_axis',(0.,0.,1.)) ;
#98775=DIRECTION('',(0.,-1.,0.)) ;
#98776=DIRECTION('center_axis',(-0.475489515607485,0.866028065754805,0.15461277396241)) ;
#98777=DIRECTION('ref_axis',(-0.823582125550541,-0.499995389303733,0.26780047264458)) ;
#98778=DIRECTION('',(-6.95778281854898E-9,-1.,-5.25180768870477E-9)) ;
#98779=DIRECTION('center_axis',(-0.475585457889948,-0.866022400932201,0.154349192829876)) ;
#98780=DIRECTION('ref_axis',(-0.823726751681711,0.500005201056575,0.267336936243893)) ;
#98781=DIRECTION('',(0.,-1.,0.)) ;
#98782=DIRECTION('center_axis',(0.,1.,0.)) ;
#98783=DIRECTION('ref_axis',(0.,0.,1.)) ;
#98784=DIRECTION('center_axis',(0.,-1.,0.)) ;
#98785=DIRECTION('ref_axis',(1.,0.,2.2577126443575E-16)) ;
#98786=DIRECTION('center_axis',(-1.42478674527368E-13,-1.,-3.7508514743183E-14)) ;
#98787=DIRECTION('ref_axis',(0.798195139400692,-1.36320876135353E-13,0.602398970315447)) ;
#98788=DIRECTION('center_axis',(0.,1.,0.)) ;
#98789=DIRECTION('ref_axis',(0.,0.,1.)) ;
#98790=DIRECTION('center_axis',(0.,1.,0.)) ;
#98791=DIRECTION('ref_axis',(0.,0.,1.)) ;
#98792=DIRECTION('',(-8.6595605623549E-17,0.70710678118655,-0.707106781186545)) ;
#98793=DIRECTION('center_axis',(0.,1.,0.)) ;
#98794=DIRECTION('ref_axis',(0.,0.,1.)) ;
#98795=DIRECTION('center_axis',(0.,1.,0.)) ;
#98796=DIRECTION('ref_axis',(0.,0.,1.)) ;
#98797=DIRECTION('center_axis',(0.,1.,0.)) ;
#98798=DIRECTION('ref_axis',(0.,0.,1.)) ;
#98799=DIRECTION('',(0.,1.,0.)) ;
#98800=DIRECTION('center_axis',(0.,1.,0.)) ;
#98801=DIRECTION('ref_axis',(0.,0.,1.)) ;
#98802=DIRECTION('',(-1.04972719113862E-16,0.515038074910058,-0.85716730070211)) ;
#98803=DIRECTION('center_axis',(0.,1.,0.)) ;
#98804=DIRECTION('ref_axis',(0.,0.,1.)) ;
#98805=DIRECTION('center_axis',(0.,1.,0.)) ;
#98806=DIRECTION('ref_axis',(0.,0.,1.)) ;
#98807=DIRECTION('center_axis',(1.,0.,-1.22464679914735E-16)) ;
#98808=DIRECTION('ref_axis',(-1.22464679914735E-16,0.,-1.)) ;
#98809=DIRECTION('center_axis',(0.,1.,0.)) ;
#98810=DIRECTION('ref_axis',(0.,0.,1.)) ;
#98811=DIRECTION('',(8.65956056235491E-17,-0.707106781186549,0.707106781186546)) ;
#98812=DIRECTION('center_axis',(0.,-1.,0.)) ;
#98813=DIRECTION('ref_axis',(0.,0.,-1.)) ;
#98814=DIRECTION('center_axis',(0.,-1.,0.)) ;
#98815=DIRECTION('ref_axis',(0.,0.,-1.)) ;
#98816=DIRECTION('',(0.,-1.,0.)) ;
#98817=DIRECTION('center_axis',(0.,-1.,0.)) ;
#98818=DIRECTION('ref_axis',(8.88178419700125E-16,0.,1.)) ;
#98819=DIRECTION('',(0.,1.,0.)) ;
#98820=DIRECTION('center_axis',(0.,1.,0.)) ;
#98821=DIRECTION('ref_axis',(0.,0.,1.)) ;
#98822=DIRECTION('center_axis',(0.,-1.,0.)) ;
#98823=DIRECTION('ref_axis',(0.,0.,-1.)) ;
#98824=DIRECTION('',(0.,1.,0.)) ;
#98825=DIRECTION('center_axis',(0.,1.,0.)) ;
#98826=DIRECTION('ref_axis',(0.,0.,1.)) ;
#98827=DIRECTION('',(0.,-1.,0.)) ;
#98828=DIRECTION('center_axis',(0.,-1.,0.)) ;
#98829=DIRECTION('ref_axis',(1.4210854715202E-14,0.,1.)) ;
#98830=DIRECTION('center_axis',(0.,-1.,0.)) ;
#98831=DIRECTION('ref_axis',(0.,0.,-1.)) ;
#98832=DIRECTION('',(0.,-1.,0.)) ;
#98833=DIRECTION('center_axis',(0.,-1.,0.)) ;
#98834=DIRECTION('ref_axis',(0.,0.,1.)) ;
#98835=DIRECTION('',(0.,1.,0.)) ;
#98836=DIRECTION('center_axis',(0.,1.,0.)) ;
#98837=DIRECTION('ref_axis',(0.,0.,1.)) ;
#98838=DIRECTION('center_axis',(0.,-1.,0.)) ;
#98839=DIRECTION('ref_axis',(0.,0.,-1.)) ;
#98840=DIRECTION('',(0.,-1.,0.)) ;
#98841=DIRECTION('center_axis',(0.,-1.,0.)) ;
#98842=DIRECTION('ref_axis',(0.,0.,1.)) ;
#98843=DIRECTION('',(0.,1.,0.)) ;
#98844=DIRECTION('center_axis',(0.,1.,0.)) ;
#98845=DIRECTION('ref_axis',(0.,0.,1.)) ;
#98846=DIRECTION('center_axis',(0.,-1.,0.)) ;
#98847=DIRECTION('ref_axis',(0.,0.,-1.)) ;
#98848=DIRECTION('',(0.,-1.,0.)) ;
#98849=DIRECTION('center_axis',(0.,-1.,0.)) ;
#98850=DIRECTION('ref_axis',(0.,0.,1.)) ;
#98851=DIRECTION('',(0.,1.,0.)) ;
#98852=DIRECTION('center_axis',(0.,1.,0.)) ;
#98853=DIRECTION('ref_axis',(0.,0.,1.)) ;
#98854=DIRECTION('center_axis',(0.,-1.,0.)) ;
#98855=DIRECTION('ref_axis',(0.,0.,-1.)) ;
#98856=DIRECTION('',(0.,-1.,0.)) ;
#98857=DIRECTION('center_axis',(0.,-1.,0.)) ;
#98858=DIRECTION('ref_axis',(0.,0.,1.)) ;
#98859=DIRECTION('',(0.,1.,0.)) ;
#98860=DIRECTION('center_axis',(0.,1.,0.)) ;
#98861=DIRECTION('ref_axis',(0.,0.,1.)) ;
#98862=DIRECTION('center_axis',(0.,1.,0.)) ;
#98863=DIRECTION('ref_axis',(0.,0.,1.)) ;
#98864=DIRECTION('center_axis',(0.,-1.,0.)) ;
#98865=DIRECTION('ref_axis',(1.77635683940025E-15,0.,1.)) ;
#98866=DIRECTION('center_axis',(0.,1.,0.)) ;
#98867=DIRECTION('ref_axis',(0.,0.,1.)) ;
#98868=DIRECTION('center_axis',(0.,-1.,0.)) ;
#98869=DIRECTION('ref_axis',(-3.5527136788005E-15,0.,1.)) ;
#98870=DIRECTION('center_axis',(0.,1.,0.)) ;
#98871=DIRECTION('ref_axis',(0.,0.,1.)) ;
#98872=DIRECTION('center_axis',(0.,-1.,0.)) ;
#98873=DIRECTION('ref_axis',(0.,0.,1.)) ;
#98874=DIRECTION('center_axis',(0.,1.,0.)) ;
#98875=DIRECTION('ref_axis',(0.,0.,1.)) ;
#98876=DIRECTION('center_axis',(0.,-1.,0.)) ;
#98877=DIRECTION('ref_axis',(0.,0.,1.)) ;
#98878=DIRECTION('center_axis',(0.,1.,0.)) ;
#98879=DIRECTION('ref_axis',(0.,0.,1.)) ;
#98880=DIRECTION('center_axis',(0.,-1.,0.)) ;
#98881=DIRECTION('ref_axis',(1.77635683940025E-15,0.,1.)) ;
#98882=DIRECTION('center_axis',(0.,1.,0.)) ;
#98883=DIRECTION('ref_axis',(0.,0.,1.)) ;
#98884=DIRECTION('center_axis',(0.,-1.,0.)) ;
#98885=DIRECTION('ref_axis',(0.,0.,1.)) ;
#98886=DIRECTION('center_axis',(0.,-1.,0.)) ;
#98887=DIRECTION('ref_axis',(0.,0.,-1.)) ;
#98888=DIRECTION('center_axis',(0.,1.,0.)) ;
#98889=DIRECTION('ref_axis',(0.,0.,1.)) ;
#98890=DIRECTION('center_axis',(0.,-1.,0.)) ;
#98891=DIRECTION('ref_axis',(0.,0.,-1.)) ;
#98892=DIRECTION('center_axis',(0.,1.,0.)) ;
#98893=DIRECTION('ref_axis',(0.,0.,1.)) ;
#98894=DIRECTION('center_axis',(0.,-1.,0.)) ;
#98895=DIRECTION('ref_axis',(0.,0.,-1.)) ;
#98896=DIRECTION('center_axis',(0.,1.,0.)) ;
#98897=DIRECTION('ref_axis',(0.,0.,1.)) ;
#98898=DIRECTION('center_axis',(0.,-1.,0.)) ;
#98899=DIRECTION('ref_axis',(0.,0.,-1.)) ;
#98900=DIRECTION('center_axis',(0.,1.,0.)) ;
#98901=DIRECTION('ref_axis',(0.,0.,1.)) ;
#98902=DIRECTION('center_axis',(0.,-1.,0.)) ;
#98903=DIRECTION('ref_axis',(0.,0.,-1.)) ;
#98904=DIRECTION('center_axis',(0.,1.,0.)) ;
#98905=DIRECTION('ref_axis',(0.,0.,1.)) ;
#98906=DIRECTION('center_axis',(0.,-1.,0.)) ;
#98907=DIRECTION('ref_axis',(0.,0.,-1.)) ;
#98908=DIRECTION('center_axis',(0.,1.,0.)) ;
#98909=DIRECTION('ref_axis',(0.,0.,1.)) ;
#98910=DIRECTION('center_axis',(0.,1.,0.)) ;
#98911=DIRECTION('ref_axis',(0.,0.,1.)) ;
#98912=DIRECTION('center_axis',(0.,1.,0.)) ;
#98913=DIRECTION('ref_axis',(0.,0.,1.)) ;
#98914=DIRECTION('center_axis',(0.,-1.,0.)) ;
#98915=DIRECTION('ref_axis',(0.,0.,-1.)) ;
#98916=DIRECTION('center_axis',(0.866025403784438,0.,-0.5)) ;
#98917=DIRECTION('ref_axis',(-0.5,0.,-0.866025403784438)) ;
#98918=DIRECTION('center_axis',(-1.66923844304129E-16,0.,-1.)) ;
#98919=DIRECTION('ref_axis',(-1.,0.,1.66923844304129E-16)) ;
#98920=DIRECTION('center_axis',(-0.866025403784439,0.,-0.5)) ;
#98921=DIRECTION('ref_axis',(-0.5,0.,0.866025403784439)) ;
#98922=DIRECTION('center_axis',(-0.866025403784439,0.,0.5)) ;
#98923=DIRECTION('ref_axis',(0.5,0.,0.866025403784439)) ;
#98924=DIRECTION('center_axis',(0.,0.,1.)) ;
#98925=DIRECTION('ref_axis',(1.,0.,0.)) ;
#98926=DIRECTION('center_axis',(0.866025403784439,0.,0.5)) ;
#98927=DIRECTION('ref_axis',(0.5,0.,-0.866025403784439)) ;
#98928=DIRECTION('',(-0.823666160229971,0.500005191429812,0.267523578465998)) ;
#98929=DIRECTION('center_axis',(0.820330601492067,0.506050349255751,-0.266403356348595)) ;
#98930=DIRECTION('ref_axis',(0.462747539860455,-0.861076590521797,-0.210741119880419)) ;
#98931=DIRECTION('center_axis',(-0.475585457889948,-0.866022400932201,0.154349192829876)) ;
#98932=DIRECTION('ref_axis',(0.876526377919256,-0.48135382912339,1.20637155219922E-16)) ;
#98933=DIRECTION('',(0.308961791614634,-0.000161847349230684,0.951074437217041)) ;
#98934=DIRECTION('center_axis',(-0.951074449673282,4.99476165283064E-9,
0.308961795661963)) ;
#98935=DIRECTION('ref_axis',(0.308961795661963,-8.41182830767154E-26,0.951074449673282)) ;
#98936=DIRECTION('',(0.308961791614634,-0.000161847349230685,0.951074437217041)) ;
#98937=DIRECTION('center_axis',(-0.475489515607485,0.866028065754805,0.15461277396241)) ;
#98938=DIRECTION('ref_axis',(-0.87656867565068,-0.481276798597245,1.5659813065563E-16)) ;
#124041=CARTESIAN_POINT('',(0.,0.,0.)) ;
#124042=CARTESIAN_POINT('Origin',(1.38777878078145E-16,-6.28125000068279,
-2.77555756156289E-16)) ;
#124043=CARTESIAN_POINT('',(-1.2293670625,-1.09375000068279,-5.21005851079475E-15)) ;
#124044=CARTESIAN_POINT('',(-1.2293670625,-0.968750000682796,-2.98084374001462E-14)) ;
#124045=CARTESIAN_POINT('',(-1.2293670625,-6.28125000068279,-7.05665556119359E-16)) ;
#124046=CARTESIAN_POINT('',(1.16918410523995,-0.819406422395167,-0.379936708431992)) ;
#124047=CARTESIAN_POINT('Ctrl Pts',(-1.2293670625,-1.09375000068279,-9.67975699595058E-15)) ;
#124048=CARTESIAN_POINT('Ctrl Pts',(-1.2293670625,-1.0846749481888,0.154589977307616)) ;
#124049=CARTESIAN_POINT('Ctrl Pts',(-1.20021118839201,-1.07468536503738,
0.307925475665665)) ;
#124050=CARTESIAN_POINT('Ctrl Pts',(-1.08420684294538,-1.05352652382332,
0.601382937533272)) ;
#124051=CARTESIAN_POINT('Ctrl Pts',(-0.996398213495616,-1.0425417450548,
0.737808020725081)) ;
#124052=CARTESIAN_POINT('Ctrl Pts',(-0.776616964406496,-1.02171673600945,
0.96566315863742)) ;
#124053=CARTESIAN_POINT('Ctrl Pts',(-0.648097680210764,-1.01268166410948,
1.05621820882725)) ;
#124054=CARTESIAN_POINT('Ctrl Pts',(-0.357410832361479,-0.992977293684764,
1.18752407058778)) ;
#124055=CARTESIAN_POINT('Ctrl Pts',(-0.196880508044035,-0.982095655942453,
1.22440775145394)) ;
#124056=CARTESIAN_POINT('Ctrl Pts',(0.124915731705902,-0.960282518003032,
1.23327661515053)) ;
#124057=CARTESIAN_POINT('Ctrl Pts',(0.283075541788596,-0.949561566892828,
1.20683758809188)) ;
#124058=CARTESIAN_POINT('Ctrl Pts',(0.579861378775666,-0.929443773081141,
1.09549036257894)) ;
#124059=CARTESIAN_POINT('Ctrl Pts',(0.715754183345007,-0.920563114801157,
1.01194688536211)) ;
#124060=CARTESIAN_POINT('Ctrl Pts',(0.952247755389101,-0.899781359138197,
0.794477416094161)) ;
#124061=CARTESIAN_POINT('Ctrl Pts',(1.0491659407666,-0.888673772908759,
0.661219760303515)) ;
#124062=CARTESIAN_POINT('Ctrl Pts',(1.18274942698846,-0.867066164473483,
0.370267045631756)) ;
#124063=CARTESIAN_POINT('Ctrl Pts',(1.22033776635663,-0.856754477438507,
0.21631311942058)) ;
#124064=CARTESIAN_POINT('Ctrl Pts',(1.23512911303773,-0.838310078143878,
-0.0893402358594326)) ;
#124065=CARTESIAN_POINT('Ctrl Pts',(1.21524070660064,-0.829287562268207,
-0.238206138425924)) ;
#124066=CARTESIAN_POINT('Ctrl Pts',(1.16918410523995,-0.819406422395166,
-0.379936708431992)) ;
#124067=CARTESIAN_POINT('',(1.16918849388564,-0.694407135956962,-0.379923189325734)) ;
#124068=CARTESIAN_POINT('',(1.16918410523995,-0.819406422395166,-0.37993670843199)) ;
#124069=CARTESIAN_POINT('Ctrl Pts',(1.16918850806102,-0.694407367007051,
-0.379923159307147)) ;
#124070=CARTESIAN_POINT('Ctrl Pts',(1.21645797241154,-0.704549055321802,
-0.234454495060375)) ;
#124071=CARTESIAN_POINT('Ctrl Pts',(1.23615258137902,-0.713735817175049,
-0.0814970379028584)) ;
#124072=CARTESIAN_POINT('Ctrl Pts',(1.21821185875717,-0.732517494081259,
0.228083416806234)) ;
#124073=CARTESIAN_POINT('Ctrl Pts',(1.17909262427295,-0.742867933316568,
0.381813608918001)) ;
#124074=CARTESIAN_POINT('Ctrl Pts',(1.0425035983168,-0.764515665918384,
0.671714573931943)) ;
#124075=CARTESIAN_POINT('Ctrl Pts',(0.944144533195031,-0.775622301867799,
0.804124149765071)) ;
#124076=CARTESIAN_POINT('Ctrl Pts',(0.705528340879558,-0.796326994915782,
1.01905539207879)) ;
#124077=CARTESIAN_POINT('Ctrl Pts',(0.569079951032635,-0.805174598185578,
1.10108618075603)) ;
#124078=CARTESIAN_POINT('Ctrl Pts',(0.271386894021466,-0.825353888413578,
1.20953938890892)) ;
#124079=CARTESIAN_POINT('Ctrl Pts',(0.112823651501299,-0.836102186417004,
1.23446116299375)) ;
#124080=CARTESIAN_POINT('Ctrl Pts',(-0.209011673067325,-0.857917973742702,
1.22239412378343)) ;
#124081=CARTESIAN_POINT('Ctrl Pts',(-0.369160526837812,-0.868773753290811,
1.18392323231963)) ;
#124082=CARTESIAN_POINT('Ctrl Pts',(-0.658474392523389,-0.888385055352298,
1.04977191270669)) ;
#124083=CARTESIAN_POINT('Ctrl Pts',(-0.786055421205409,-0.897487203807662,
0.957987835975483)) ;
#124084=CARTESIAN_POINT('Ctrl Pts',(-1.00367155178044,-0.918368881220496,
0.727917342783409)) ;
#124085=CARTESIAN_POINT('Ctrl Pts',(-1.09020270986942,-0.929369371550939,
0.590487070832282)) ;
#124086=CARTESIAN_POINT('Ctrl Pts',(-1.2017840793143,-0.950226809738017,
0.299610285508617)) ;
#124087=CARTESIAN_POINT('Ctrl Pts',(-1.22936706250001,-0.959922721618476,
0.150369253637278)) ;
#124088=CARTESIAN_POINT('Ctrl Pts',(-1.2293670625,-0.968750000682796,-5.94663207564849E-14)) ;
#124089=CARTESIAN_POINT('Origin',(1.38777878078145E-16,-6.28125000068279,
-2.77555756156289E-16)) ;
#124090=CARTESIAN_POINT('',(-1.2293670625,-1.59375000068279,2.42108516417716E-14)) ;
#124091=CARTESIAN_POINT('',(-1.2293670625,-1.46875000068279,4.41765678087653E-15)) ;
#124092=CARTESIAN_POINT('',(-1.2293670625,-6.28125000068279,-7.05665556119359E-16)) ;
#124093=CARTESIAN_POINT('Ctrl Pts',(-1.2293670625,-1.59375000068279,4.91273688396627E-14)) ;
#124094=CARTESIAN_POINT('Ctrl Pts',(-1.2293670625,-1.5929636944515,0.0133944197603256)) ;
#124095=CARTESIAN_POINT('Ctrl Pts',(-1.22914815761871,-1.59216952410361,
0.0267964168859271)) ;
#124096=CARTESIAN_POINT('Ctrl Pts',(-1.22337688007584,-1.58161879139812,
0.203191982006123)) ;
#124097=CARTESIAN_POINT('Ctrl Pts',(-1.18566753703356,-1.57093214183561,
0.36346338702498)) ;
#124098=CARTESIAN_POINT('Ctrl Pts',(-1.05128310495245,-1.54914312506858,
0.657043895518347)) ;
#124099=CARTESIAN_POINT('Ctrl Pts',(-0.957014484116075,-1.53825707637603,
0.788057472633634)) ;
#124100=CARTESIAN_POINT('Ctrl Pts',(-0.726080978284878,-1.51773530910495,
1.00430824684218)) ;
#124101=CARTESIAN_POINT('Ctrl Pts',(-0.592534031366209,-1.50891525112215,
1.08845244229616)) ;
#124102=CARTESIAN_POINT('Ctrl Pts',(-0.293706456717641,-1.4886590569821,
1.20501927343027)) ;
#124103=CARTESIAN_POINT('Ctrl Pts',(-0.130245411804608,-1.47757875870646,
1.23343243303519)) ;
#124104=CARTESIAN_POINT('Ctrl Pts',(0.191877553061588,-1.45574347352245,
1.22453704189747)) ;
#124105=CARTESIAN_POINT('Ctrl Pts',(0.347535237170195,-1.44519213041965,
1.18976666575577)) ;
#124106=CARTESIAN_POINT('Ctrl Pts',(0.639126244266634,-1.42542647105511,
1.06231616683244)) ;
#124107=CARTESIAN_POINT('Ctrl Pts',(0.771929174362773,-1.41620378837636,
0.970120107315155)) ;
#124108=CARTESIAN_POINT('Ctrl Pts',(0.996185419970736,-1.39500206676428,
0.738431458301724)) ;
#124109=CARTESIAN_POINT('Ctrl Pts',(1.08483303727253,-1.38391015640713,
0.600665820172445)) ;
#124110=CARTESIAN_POINT('Ctrl Pts',(1.20134026294244,-1.36255891131156,
0.304221171309325)) ;
#124111=CARTESIAN_POINT('Ctrl Pts',(1.23021641354854,-1.35254167696737,
0.149272401123027)) ;
#124112=CARTESIAN_POINT('Ctrl Pts',(1.22844108996505,-1.33374566651196,
-0.169885317488781)) ;
#124113=CARTESIAN_POINT('Ctrl Pts',(1.19510722167321,-1.32315253950266,
-0.33108978383975)) ;
#124114=CARTESIAN_POINT('Ctrl Pts',(1.06861176256678,-1.30140166463955,
-0.628575260556984)) ;
#124115=CARTESIAN_POINT('Ctrl Pts',(0.977633222956603,-1.29046118528742,
-0.76241557199597)) ;
#124116=CARTESIAN_POINT('Ctrl Pts',(0.752425302092438,-1.26978135739856,
-0.984664515160361)) ;
#124117=CARTESIAN_POINT('Ctrl Pts',(0.621501524548423,-1.26087882883529,
-1.0721180183845)) ;
#124118=CARTESIAN_POINT('Ctrl Pts',(0.325900396799594,-1.24084134120136,
-1.19677560672971)) ;
#124119=CARTESIAN_POINT('Ctrl Pts',(0.162802692597181,-1.22978567217883,
-1.22961794504459)) ;
#124120=CARTESIAN_POINT('Ctrl Pts',(-0.160283283818217,-1.2078851087188,
-1.22912292604001)) ;
#124121=CARTESIAN_POINT('Ctrl Pts',(-0.317178287315828,-1.19724989322978,
-1.19826854858965)) ;
#124122=CARTESIAN_POINT('Ctrl Pts',(-0.611257629180353,-1.17731556070243,
-1.07843535840023)) ;
#124123=CARTESIAN_POINT('Ctrl Pts',(-0.745523661530749,-1.16828825891483,
-0.990383019442521)) ;
#124124=CARTESIAN_POINT('Ctrl Pts',(-0.975660261061792,-1.14728319141039,
-0.7654393203204)) ;
#124125=CARTESIAN_POINT('Ctrl Pts',(-1.06827259754044,-1.13617936197068,
-0.62975967695568)) ;
#124126=CARTESIAN_POINT('Ctrl Pts',(-1.19291445872554,-1.11470249565326,
-0.335871653611875)) ;
#124127=CARTESIAN_POINT('Ctrl Pts',(-1.22596595845213,-1.10451088909497,
-0.181343905866327)) ;
#124128=CARTESIAN_POINT('Ctrl Pts',(-1.22928414193443,-1.09472088788474,
-0.0164908103436252)) ;
#124129=CARTESIAN_POINT('Ctrl Pts',(-1.2293670625,-1.09423394389032,-0.00824378366076975)) ;
#124130=CARTESIAN_POINT('Ctrl Pts',(-1.2293670625,-1.09375000068279,-9.71445146547014E-15)) ;
#124131=CARTESIAN_POINT('Ctrl Pts',(-1.2293670625,-0.968750000682796,-5.89112092441731E-14)) ;
#124132=CARTESIAN_POINT('Ctrl Pts',(-1.2293670625,-0.969561252441858,-0.0138193570899708)) ;
#124133=CARTESIAN_POINT('Ctrl Pts',(-1.2291340479447,-0.970380907670849,
-0.0276473329945444)) ;
#124134=CARTESIAN_POINT('Ctrl Pts',(-1.22337520926784,-0.980590330322463,
-0.198235996140464)) ;
#124135=CARTESIAN_POINT('Ctrl Pts',(-1.18813428765872,-0.990840862008632,
-0.352503447128259)) ;
#124136=CARTESIAN_POINT('Ctrl Pts',(-1.0591708524137,-1.01238302768322,
-0.645008757588703)) ;
#124137=CARTESIAN_POINT('Ctrl Pts',(-0.964473899961518,-1.02348989465029,
-0.779536590453002)) ;
#124138=CARTESIAN_POINT('Ctrl Pts',(-0.731256601296687,-1.04438813821597,
-1.00088194299678)) ;
#124139=CARTESIAN_POINT('Ctrl Pts',(-0.596208734201048,-1.05333565845826,
-1.08675312767868)) ;
#124140=CARTESIAN_POINT('Ctrl Pts',(-0.300819820295893,-1.0733587610582,
-1.20250729295855)) ;
#124141=CARTESIAN_POINT('Ctrl Pts',(-0.143301720801929,-1.08403621345754,
-1.23124582846075)) ;
#124142=CARTESIAN_POINT('Ctrl Pts',(0.178373476902107,-1.10584114649424,
-1.22724221806317)) ;
#124143=CARTESIAN_POINT('Ctrl Pts',(0.339453479583223,-1.1167600444916,
-1.19278259194041)) ;
#124144=CARTESIAN_POINT('Ctrl Pts',(0.632211559049604,-1.13660481450894,
-1.06582143468517)) ;
#124145=CARTESIAN_POINT('Ctrl Pts',(0.7621669073982,-1.14555401570759,-0.97712690087377)) ;
#124146=CARTESIAN_POINT('Ctrl Pts',(0.98521007958537,-1.16629229695877,
-0.752632409264716)) ;
#124147=CARTESIAN_POINT('Ctrl Pts',(1.07492981302683,-1.17725129431447,
-0.617749878782074)) ;
#124148=CARTESIAN_POINT('Ctrl Pts',(1.19848488575403,-1.19899347881046,
-0.318714806209338)) ;
#124149=CARTESIAN_POINT('Ctrl Pts',(1.23011615353584,-1.20949855073417,
-0.157162351188974)) ;
#124150=CARTESIAN_POINT('Ctrl Pts',(1.22862156582599,-1.22829404501319,
0.162148657491748)) ;
#124151=CARTESIAN_POINT('Ctrl Pts',(1.19805319996093,-1.23841662568408,
0.316934214189202)) ;
#124152=CARTESIAN_POINT('Ctrl Pts',(1.07832719948975,-1.25981447009513,
0.612314303705971)) ;
#124153=CARTESIAN_POINT('Ctrl Pts',(0.988094145778355,-1.27091209897793,
0.749262002550019)) ;
#124154=CARTESIAN_POINT('Ctrl Pts',(0.761482650580558,-1.29203619338474,
0.978268498434431)) ;
#124155=CARTESIAN_POINT('Ctrl Pts',(0.628097914878412,-1.30117403252555,
1.06880791258277)) ;
#124156=CARTESIAN_POINT('Ctrl Pts',(0.335512092244417,-1.32100712601724,
1.19323354512822)) ;
#124157=CARTESIAN_POINT('Ctrl Pts',(0.179351679657468,-1.33159254685088,
1.22645458408494)) ;
#124158=CARTESIAN_POINT('Ctrl Pts',(-0.143179062758288,-1.35345547346396,
1.23202141102484)) ;
#124159=CARTESIAN_POINT('Ctrl Pts',(-0.306509769412905,-1.36452693668793,
1.20185074800083)) ;
#124160=CARTESIAN_POINT('Ctrl Pts',(-0.604066552363513,-1.38469698950258,
1.08206937457938)) ;
#124161=CARTESIAN_POINT('Ctrl Pts',(-0.736568263154353,-1.39354235236009,
0.9966154167158)) ;
#124162=CARTESIAN_POINT('Ctrl Pts',(-0.965244170093328,-1.41412704291671,
0.777989343568323)) ;
#124163=CARTESIAN_POINT('Ctrl Pts',(-1.05822258321062,-1.42503550116704,
0.645849126608738)) ;
#124164=CARTESIAN_POINT('Ctrl Pts',(-1.18950334941557,-1.44681140540772,
0.350700082554891)) ;
#124165=CARTESIAN_POINT('Ctrl Pts',(-1.22548651319292,-1.45746205873105,
0.190045249358232)) ;
#124166=CARTESIAN_POINT('Ctrl Pts',(-1.22926817372685,-1.46768945647037,
0.0180088632755795)) ;
#124167=CARTESIAN_POINT('Ctrl Pts',(-1.2293670625,-1.46822151063544,0.00900262169078512)) ;
#124168=CARTESIAN_POINT('Ctrl Pts',(-1.2293670625,-1.46875000068279,9.54097911787242E-15)) ;
#124169=CARTESIAN_POINT('Origin',(1.38777878078145E-16,-6.28125000068279,
-2.77555756156289E-16)) ;
#124170=CARTESIAN_POINT('',(-1.2293670625,-2.09375000068277,1.96156642580576E-13)) ;
#124171=CARTESIAN_POINT('',(-1.2293670625,-1.96875000068277,1.76519572832522E-13)) ;
#124172=CARTESIAN_POINT('',(-1.2293670625,-6.28125000068279,-7.05665556119359E-16)) ;
#124173=CARTESIAN_POINT('Ctrl Pts',(-1.2293670625,-2.09375000068277,3.93018950717272E-13)) ;
#124174=CARTESIAN_POINT('Ctrl Pts',(-1.2293670625,-2.09165438781884,0.0356979472348365)) ;
#124175=CARTESIAN_POINT('Ctrl Pts',(-1.22781227856084,-2.08950396001902,
0.0714319905826287)) ;
#124176=CARTESIAN_POINT('Ctrl Pts',(-1.21048122524801,-2.0772828419258,
0.269607879191005)) ;
#124177=CARTESIAN_POINT('Ctrl Pts',(-1.16407025798557,-2.06643292732197,
0.427636555381604)) ;
#124178=CARTESIAN_POINT('Ctrl Pts',(-1.01421336879494,-2.04461684769803,
0.712745041802709)) ;
#124179=CARTESIAN_POINT('Ctrl Pts',(-0.913596365833781,-2.03386263496667,
0.837847604645138)) ;
#124180=CARTESIAN_POINT('Ctrl Pts',(-0.671280967314773,-2.01366982229743,
1.04192342679273)) ;
#124181=CARTESIAN_POINT('Ctrl Pts',(-0.532242729905873,-2.00482837156033,
1.11934866326663)) ;
#124182=CARTESIAN_POINT('Ctrl Pts',(-0.227050909601382,-1.98414077347199,
1.21921468555743)) ;
#124183=CARTESIAN_POINT('Ctrl Pts',(-0.0632066373057889,-1.97303449791407,
1.23856003380864)) ;
#124184=CARTESIAN_POINT('Ctrl Pts',(0.256275879686575,-1.95137819696474,
1.21258984202624)) ;
#124185=CARTESIAN_POINT('Ctrl Pts',(0.409093928059733,-1.94101934015713,
1.16992076791325)) ;
#124186=CARTESIAN_POINT('Ctrl Pts',(0.695384673063911,-1.92161296202043,
1.02678847829774)) ;
#124187=CARTESIAN_POINT('Ctrl Pts',(0.825134773353636,-1.91179643974479,
0.925760910432755)) ;
#124188=CARTESIAN_POINT('Ctrl Pts',(1.03673917815347,-1.89020351767688,
0.680103770640548)) ;
#124189=CARTESIAN_POINT('Ctrl Pts',(1.11694520626755,-1.87916265408012,
0.53833394036141)) ;
#124190=CARTESIAN_POINT('Ctrl Pts',(1.21629298572484,-1.85811584366874,
0.2371682066349)) ;
#124191=CARTESIAN_POINT('Ctrl Pts',(1.23651862738949,-1.84876701661882,
0.0813339504507454)) ;
#124192=CARTESIAN_POINT('Ctrl Pts',(1.21729932128853,-1.82943313601169,
-0.236914888266518)) ;
#124193=CARTESIAN_POINT('Ctrl Pts',(1.17516767052112,-1.81865968229379,
-0.396111747637677)) ;
#124194=CARTESIAN_POINT('Ctrl Pts',(1.03288359615056,-1.79684870117668,
-0.685505549659799)) ;
#124195=CARTESIAN_POINT('Ctrl Pts',(0.935356034691252,-1.78602568611029,
-0.81356382330911)) ;
#124196=CARTESIAN_POINT('Ctrl Pts',(0.698641389678176,-1.76566863202775,
-1.02367103037446)) ;
#124197=CARTESIAN_POINT('Ctrl Pts',(0.562350489766241,-1.75686924288746,
-1.10442891361411)) ;
#124198=CARTESIAN_POINT('Ctrl Pts',(0.260280297711559,-1.73639324611448,
-1.21261626569671)) ;
#124199=CARTESIAN_POINT('Ctrl Pts',(0.0965657576394018,-1.72529576452781,
-1.23646516205919)) ;
#124200=CARTESIAN_POINT('Ctrl Pts',(-0.224340566425014,-1.70354295002045,
-1.21895446149861)) ;
#124201=CARTESIAN_POINT('Ctrl Pts',(-0.378620423336193,-1.69308500370419,
-1.18018834916704)) ;
#124202=CARTESIAN_POINT('Ctrl Pts',(-0.667579897397263,-1.67349772427702,
-1.04486279772397)) ;
#124203=CARTESIAN_POINT('Ctrl Pts',(-0.798859430521799,-1.66400913970839,
-0.948283314454632)) ;
#124204=CARTESIAN_POINT('Ctrl Pts',(-1.01685635677711,-1.64260846532705,
-0.709591762953443)) ;
#124205=CARTESIAN_POINT('Ctrl Pts',(-1.10131027098922,-1.63153764939205,
-0.569764224464767)) ;
#124206=CARTESIAN_POINT('Ctrl Pts',(-1.20468360637947,-1.61123179889717,
-0.283544609526032)) ;
#124207=CARTESIAN_POINT('Ctrl Pts',(-1.2293670625,-1.60210052180872,-0.142247868232065)) ;
#124208=CARTESIAN_POINT('Ctrl Pts',(-1.2293670625,-1.59375000068279,4.88498130835069E-14)) ;
#124209=CARTESIAN_POINT('Ctrl Pts',(-1.2293670625,-1.46875000068279,9.22872889219661E-15)) ;
#124210=CARTESIAN_POINT('Ctrl Pts',(-1.2293670625,-1.47736724240036,-0.146791349411587)) ;
#124211=CARTESIAN_POINT('Ctrl Pts',(-1.20307951446642,-1.48681290739968,
-0.292517443166858)) ;
#124212=CARTESIAN_POINT('Ctrl Pts',(-1.09493092752208,-1.50747090916634,
-0.58197882480792)) ;
#124213=CARTESIAN_POINT('Ctrl Pts',(-1.00882144120501,-1.51855107489725,
-0.721009788420243)) ;
#124214=CARTESIAN_POINT('Ctrl Pts',(-0.788347960357798,-1.53987430492733,
-0.956952266163614)) ;
#124215=CARTESIAN_POINT('Ctrl Pts',(-0.656469261544164,-1.54925086493719,
-1.05180073591998)) ;
#124216=CARTESIAN_POINT('Ctrl Pts',(-0.366470758871749,-1.56890857549942,
-1.18403844371561)) ;
#124217=CARTESIAN_POINT('Ctrl Pts',(-0.211638887418654,-1.57940394042988,
-1.22124454314158)) ;
#124218=CARTESIAN_POINT('Ctrl Pts',(0.109771023084182,-1.60119089082539,
-1.23538629411922)) ;
#124219=CARTESIAN_POINT('Ctrl Pts',(0.273400911000042,-1.61228263421834,
-1.20974993006314)) ;
#124220=CARTESIAN_POINT('Ctrl Pts',(0.574211105371675,-1.63267322134425,
-1.09827509239713)) ;
#124221=CARTESIAN_POINT('Ctrl Pts',(0.709422123302591,-1.64147300103867,
-1.01619317767247)) ;
#124222=CARTESIAN_POINT('Ctrl Pts',(0.943886318187304,-1.66189478869789,
-0.803683961406093)) ;
#124223=CARTESIAN_POINT('Ctrl Pts',(1.04015319533478,-1.67274330845377,
-0.674463368898782)) ;
#124224=CARTESIAN_POINT('Ctrl Pts',(1.17937093493386,-1.69454773917046,
-0.383410801185453)) ;
#124225=CARTESIAN_POINT('Ctrl Pts',(1.21978105472352,-1.70528833345974,
-0.223779762982546)) ;
#124226=CARTESIAN_POINT('Ctrl Pts',(1.23557210196305,-1.72451804821813,
0.0946739573331135)) ;
#124227=CARTESIAN_POINT('Ctrl Pts',(1.21365982179292,-1.73397712347788,
0.250319514127987)) ;
#124228=CARTESIAN_POINT('Ctrl Pts',(1.11097892959094,-1.75508450037914,
0.550592600830559)) ;
#124229=CARTESIAN_POINT('Ctrl Pts',(1.0291181553708,-1.76613804226454,0.691623032698593)) ;
#124230=CARTESIAN_POINT('Ctrl Pts',(0.815016630588374,-1.78765717379843,
0.934581466649517)) ;
#124231=CARTESIAN_POINT('Ctrl Pts',(0.684671650277794,-1.79733915025667,
1.03387490725552)) ;
#124232=CARTESIAN_POINT('Ctrl Pts',(0.397340687297885,-1.81681604015015,
1.1739852240539)) ;
#124233=CARTESIAN_POINT('Ctrl Pts',(0.243945652517922,-1.82721400830378,
1.21515064916355)) ;
#124234=CARTESIAN_POINT('Ctrl Pts',(-0.0761134399203039,-1.84890939274191,
1.23785648021424)) ;
#124235=CARTESIAN_POINT('Ctrl Pts',(-0.239921769047805,-1.86001323187211,
1.21677070536761)) ;
#124236=CARTESIAN_POINT('Ctrl Pts',(-0.543915824845551,-1.88061963882401,
1.11368192566813)) ;
#124237=CARTESIAN_POINT('Ctrl Pts',(-0.681888322082539,-1.88943761756165,
1.03496849326193)) ;
#124238=CARTESIAN_POINT('Ctrl Pts',(-0.92205026961941,-1.90969407799152,
0.828565160848998)) ;
#124239=CARTESIAN_POINT('Ctrl Pts',(-1.02148790594684,-1.9204756400724,
0.702315804868243)) ;
#124240=CARTESIAN_POINT('Ctrl Pts',(-1.16844390552385,-1.94229166039066,
0.415533499296891)) ;
#124241=CARTESIAN_POINT('Ctrl Pts',(-1.21321088382915,-1.95311308808705,
0.257040928989308)) ;
#124242=CARTESIAN_POINT('Ctrl Pts',(-1.22815948864037,-1.96501358188157,
0.0629512428882878)) ;
#124243=CARTESIAN_POINT('Ctrl Pts',(-1.2293670625,-1.96690316013386,0.031460207942469)) ;
#124244=CARTESIAN_POINT('Ctrl Pts',(-1.2293670625,-1.96875000068277,3.53744811221163E-13)) ;
#124245=CARTESIAN_POINT('Origin',(1.38777878078145E-16,-6.28125000068279,
-2.77555756156289E-16)) ;
#124246=CARTESIAN_POINT('',(-1.2293670625,-2.59375000068278,7.81954462141675E-14)) ;
#124247=CARTESIAN_POINT('',(-1.2293670625,-2.46875000068278,1.17469585710279E-13)) ;
#124248=CARTESIAN_POINT('',(-1.2293670625,-6.28125000068279,-7.05665556119359E-16)) ;
#124249=CARTESIAN_POINT('Ctrl Pts',(-1.2293670625,-2.59375000068278,1.57096557984454E-13)) ;
#124250=CARTESIAN_POINT('Ctrl Pts',(-1.2293670625,-2.59041798638127,0.0567595631653337)) ;
#124251=CARTESIAN_POINT('Ctrl Pts',(-1.22543686828171,-2.58695022597981,
0.113562409472403)) ;
#124252=CARTESIAN_POINT('Ctrl Pts',(-1.19480516907715,-2.57303397011835,
0.332935176876669)) ;
#124253=CARTESIAN_POINT('Ctrl Pts',(-1.1395877039601,-2.56196442677115,
0.489620709083913)) ;
#124254=CARTESIAN_POINT('Ctrl Pts',(-0.974041076411476,-2.5400962334137,
0.76655845795135)) ;
#124255=CARTESIAN_POINT('Ctrl Pts',(-0.867410782333212,-2.52950410624931,
0.885428181176129)) ;
#124256=CARTESIAN_POINT('Ctrl Pts',(-0.613787858855096,-2.50965757318927,
1.0770768627525)) ;
#124257=CARTESIAN_POINT('Ctrl Pts',(-0.46891377075706,-2.50053558267458,
1.14758762858906)) ;
#124258=CARTESIAN_POINT('Ctrl Pts',(-0.157513148493988,-2.47942711747584,
1.23001001946445)) ;
#124259=CARTESIAN_POINT('Ctrl Pts',(0.006218152925851,-2.46832849971186,
1.24003667142442)) ;
#124260=CARTESIAN_POINT('Ctrl Pts',(0.322046623598325,-2.4469198903343,
1.19669326815554)) ;
#124261=CARTESIAN_POINT('Ctrl Pts',(0.471515827620829,-2.43678803681242,
1.14607411866743)) ;
#124262=CARTESIAN_POINT('Ctrl Pts',(0.749151391346744,-2.4179683549754,
0.988261200208687)) ;
#124263=CARTESIAN_POINT('Ctrl Pts',(0.873466868907703,-2.40749203866311,
0.880341666361781)) ;
#124264=CARTESIAN_POINT('Ctrl Pts',(1.07120344959392,-2.38575349716913,
0.624197364495544)) ;
#124265=CARTESIAN_POINT('Ctrl Pts',(1.14345926894784,-2.3747909469172,0.479171516312729)) ;
#124266=CARTESIAN_POINT('Ctrl Pts',(1.22695710483627,-2.35404111192044,
0.173913673680809)) ;
#124267=CARTESIAN_POINT('Ctrl Pts',(1.23910029772179,-2.34508162647748,
0.0170642397129778)) ;
#124268=CARTESIAN_POINT('Ctrl Pts',(1.20331046761246,-2.32525541988233,
-0.30000418356211)) ;
#124269=CARTESIAN_POINT('Ctrl Pts',(1.15292816679629,-2.31434132547231,
-0.456833287205966)) ;
#124270=CARTESIAN_POINT('Ctrl Pts',(0.996107159246821,-2.29253501246639,
-0.737754667491894)) ;
#124271=CARTESIAN_POINT('Ctrl Pts',(0.892680168271379,-2.28185165155821,
-0.860027949842806)) ;
#124272=CARTESIAN_POINT('Ctrl Pts',(0.645153465138463,-2.26181589338037,
-1.0584196619051)) ;
#124273=CARTESIAN_POINT('Ctrl Pts',(0.503476137496918,-2.25287841201838,
-1.13269166401237)) ;
#124274=CARTESIAN_POINT('Ctrl Pts',(0.195404224196466,-2.23199558521684,
-1.2246286865075)) ;
#124275=CARTESIAN_POINT('Ctrl Pts',(0.0315475709482201,-2.22088847040912,
-1.23971560736718)) ;
#124276=CARTESIAN_POINT('Ctrl Pts',(-0.286383953719449,-2.19933730434125,
-1.20578422735289)) ;
#124277=CARTESIAN_POINT('Ctrl Pts',(-0.437726039859254,-2.18907849645844,
-1.15946100120441)) ;
#124278=CARTESIAN_POINT('Ctrl Pts',(-0.721421918168738,-2.16984801281072,
-1.00890347709829)) ;
#124279=CARTESIAN_POINT('Ctrl Pts',(-0.849691297930594,-2.15966018389652,
-0.903548341897603)) ;
#124280=CARTESIAN_POINT('Ctrl Pts',(-1.05503584224954,-2.13788960898763,
-0.651250823162222)) ;
#124281=CARTESIAN_POINT('Ctrl Pts',(-1.13112248596896,-2.12688577801174,
-0.507733501436846)) ;
#124282=CARTESIAN_POINT('Ctrl Pts',(-1.21192352861261,-2.10835460046965,
-0.238712628313484)) ;
#124283=CARTESIAN_POINT('Ctrl Pts',(-1.2293670625,-2.10077062207742,-0.119593545360066)) ;
#124284=CARTESIAN_POINT('Ctrl Pts',(-1.2293670625,-2.09375000068277,3.92845478369708E-13)) ;
#124285=CARTESIAN_POINT('Ctrl Pts',(-1.2293670625,-1.96875000068277,3.53744811221163E-13)) ;
#124286=CARTESIAN_POINT('Ctrl Pts',(-1.2293670625,-1.97602011811598,-0.123843612999709)) ;
#124287=CARTESIAN_POINT('Ctrl Pts',(-1.21066132790823,-1.98389183184118,
-0.247135423133918)) ;
#124288=CARTESIAN_POINT('Ctrl Pts',(-1.12578541802853,-2.00275804813483,
-0.519510924931424)) ;
#124289=CARTESIAN_POINT('Ctrl Pts',(-1.04811519801998,-2.01377702882892,
-0.66237203799655)) ;
#124290=CARTESIAN_POINT('Ctrl Pts',(-0.840356495119533,-2.03548032780585,
-0.912129722381499)) ;
#124291=CARTESIAN_POINT('Ctrl Pts',(-0.711517533433462,-2.0455193870648,
-1.0158192466044)) ;
#124292=CARTESIAN_POINT('Ctrl Pts',(-0.426823083637583,-2.06481755943875,
-1.16353821348196)) ;
#124293=CARTESIAN_POINT('Ctrl Pts',(-0.274907102661338,-2.07511526910376,
-1.20847145320079)) ;
#124294=CARTESIAN_POINT('Ctrl Pts',(0.0436397000272458,-2.09670814213611,
-1.23936975273838)) ;
#124295=CARTESIAN_POINT('Ctrl Pts',(0.207504304544632,-2.10781579592505,
-1.22265811063854)) ;
#124296=CARTESIAN_POINT('Ctrl Pts',(0.514485845843513,-2.12862471125114,
-1.1276881894575)) ;
#124297=CARTESIAN_POINT('Ctrl Pts',(0.65515090648707,-2.13751912062421,
-1.05221248572423)) ;
#124298=CARTESIAN_POINT('Ctrl Pts',(0.900698625889017,-2.15761502660094,
-0.851653612593324)) ;
#124299=CARTESIAN_POINT('Ctrl Pts',(1.00306605051807,-2.16832607035337,
-0.72829702287968)) ;
#124300=CARTESIAN_POINT('Ctrl Pts',(1.15725220582521,-2.19013775064452,
-0.445762980333208)) ;
#124301=CARTESIAN_POINT('Ctrl Pts',(1.20612781607305,-2.20102827364389,
-0.288465518264877)) ;
#124302=CARTESIAN_POINT('Ctrl Pts',(1.23887181053964,-2.22076540786069,
0.0288441058375796)) ;
#124303=CARTESIAN_POINT('Ctrl Pts',(1.22525026400788,-2.22977878149898,
0.185494142032774)) ;
#124304=CARTESIAN_POINT('Ctrl Pts',(1.13887075927967,-2.25058368608936,
0.490026341418299)) ;
#124305=CARTESIAN_POINT('Ctrl Pts',(1.06516063862746,-2.26156267277276,
0.634492536550117)) ;
#124306=CARTESIAN_POINT('Ctrl Pts',(0.86483519491506,-2.28328258411032,
0.888824800207864)) ;
#124307=CARTESIAN_POINT('Ctrl Pts',(0.739459526525195,-2.29362532344838,
0.995539248251014)) ;
#124308=CARTESIAN_POINT('Ctrl Pts',(0.460128937266179,-2.31255990353838,
1.15071369555177)) ;
#124309=CARTESIAN_POINT('Ctrl Pts',(0.310012498096698,-2.32273563025639,
1.1998871679237)) ;
#124310=CARTESIAN_POINT('Ctrl Pts',(-0.00655816362446758,-2.34419454946894,
1.24005672079214)) ;
#124311=CARTESIAN_POINT('Ctrl Pts',(-0.170348886917707,-2.35529719517782,
1.22832051933773)) ;
#124312=CARTESIAN_POINT('Ctrl Pts',(-0.480636390556873,-2.37633020700859,
1.14267145379631)) ;
#124313=CARTESIAN_POINT('Ctrl Pts',(-0.624422912529161,-2.38538137805601,
1.07088728044485)) ;
#124314=CARTESIAN_POINT('Ctrl Pts',(-0.875997192095689,-2.40529216881394,
0.876961208950336)) ;
#124315=CARTESIAN_POINT('Ctrl Pts',(-0.981561473325557,-2.41591595614751,
0.756936704295497)) ;
#124316=CARTESIAN_POINT('Ctrl Pts',(-1.14450005928456,-2.43780819134319,
0.478083658583261)) ;
#124317=CARTESIAN_POINT('Ctrl Pts',(-1.19817685059442,-2.44886780965977,
0.32067768696166)) ;
#124318=CARTESIAN_POINT('Ctrl Pts',(-1.2260031200219,-2.46246809002492,
0.105067723177115)) ;
#124319=CARTESIAN_POINT('Ctrl Pts',(-1.2293670625,-2.46566738973036,0.0525110744537505)) ;
#124320=CARTESIAN_POINT('Ctrl Pts',(-1.2293670625,-2.46875000068278,2.35644836976677E-13)) ;
#124321=CARTESIAN_POINT('Origin',(1.38777878078145E-16,-6.28125000068279,
-2.77555756156289E-16)) ;
#124322=CARTESIAN_POINT('',(-1.2293670625,-3.09375000068279,-4.22221717098752E-16)) ;
#124323=CARTESIAN_POINT('',(-1.2293670625,-2.96875000068279,-4.74263421378056E-16)) ;
#124324=CARTESIAN_POINT('',(-1.2293670625,-6.28125000068279,-7.05665556119359E-16)) ;
#124325=CARTESIAN_POINT('Ctrl Pts',(-1.2293670625,-3.09375000068279,-1.38777878078145E-16)) ;
#124326=CARTESIAN_POINT('Ctrl Pts',(-1.2293670625,-3.08907858841676,0.0795756847333051)) ;
#124327=CARTESIAN_POINT('Ctrl Pts',(-1.22164306954691,-3.08414664976013,
0.15912988543831)) ;
#124328=CARTESIAN_POINT('Ctrl Pts',(-1.17458248654693,-3.06852479441537,
0.398071653875583)) ;
#124329=CARTESIAN_POINT('Ctrl Pts',(-1.11125235594702,-3.05742160331921,
0.550646512753655)) ;
#124330=CARTESIAN_POINT('Ctrl Pts',(-0.932081198075618,-3.03571849836161,
0.816905918913092)) ;
#124331=CARTESIAN_POINT('Ctrl Pts',(-0.819942382837346,-3.02531265364806,
0.92942204711778)) ;
#124332=CARTESIAN_POINT('Ctrl Pts',(-0.555366920714295,-3.00582142925331,
1.10869473312039)) ;
#124333=CARTESIAN_POINT('Ctrl Pts',(-0.404448494324175,-2.99616576788673,
1.17221119465974)) ;
#124334=CARTESIAN_POINT('Ctrl Pts',(-0.0872134952455146,-2.97466181619515,
1.23686382378819)) ;
#124335=CARTESIAN_POINT('Ctrl Pts',(0.075888549641947,-2.96360585293686,
1.23761013237613)) ;
#124336=CARTESIAN_POINT('Ctrl Pts',(0.387454086296202,-2.94248620892396,
1.17707813246554)) ;
#124337=CARTESIAN_POINT('Ctrl Pts',(0.533342525856703,-2.93300347345133,
1.11854812003175)) ;
#124338=CARTESIAN_POINT('Ctrl Pts',(0.801619005635154,-2.91379501973696,
0.946229105745676)) ;
#124339=CARTESIAN_POINT('Ctrl Pts',(0.91990801488037,-2.9030612584997,0.831677863708403)) ;
#124340=CARTESIAN_POINT('Ctrl Pts',(1.102959175131,-2.88125847403389,0.565960576449154)) ;
#124341=CARTESIAN_POINT('Ctrl Pts',(1.16706618916963,-2.87040491535142,
0.418086642171035)) ;
#124342=CARTESIAN_POINT('Ctrl Pts',(1.23452333449516,-2.84997005106801,
0.108933105695769)) ;
#124343=CARTESIAN_POINT('Ctrl Pts',(1.23834432366122,-2.84116898791691,
-0.0491495692642937)) ;
#124344=CARTESIAN_POINT('Ctrl Pts',(1.18518353494756,-2.82079580679762,
-0.365506362451576)) ;
#124345=CARTESIAN_POINT('Ctrl Pts',(1.1258936245669,-2.80970538121382,-0.520196388040076)) ;
#124346=CARTESIAN_POINT('Ctrl Pts',(0.953484360932666,-2.78791180440425,
-0.791900928345222)) ;
#124347=CARTESIAN_POINT('Ctrl Pts',(0.844066384664019,-2.77740899183833,
-0.907639743180857)) ;
#124348=CARTESIAN_POINT('Ctrl Pts',(0.58498249902388,-2.75773710547782,
-1.09316049841969)) ;
#124349=CARTESIAN_POINT('Ctrl Pts',(0.437143185563796,-2.74838199580304,
-1.16022547474248)) ;
#124350=CARTESIAN_POINT('Ctrl Pts',(0.122806801786795,-2.7270745283695,
-1.23389875445401)) ;
#124351=CARTESIAN_POINT('Ctrl Pts',(-0.0406776909787178,-2.71599264066807,
-1.2393264481315)) ;
#124352=CARTESIAN_POINT('Ctrl Pts',(-0.354503158377584,-2.69471980598674,
-1.18744927179352)) ;
#124353=CARTESIAN_POINT('Ctrl Pts',(-0.502179089971365,-2.68490265480334,
-1.13290771502913)) ;
#124354=CARTESIAN_POINT('Ctrl Pts',(-0.775238664101213,-2.6659645740121,
-0.967955918775394)) ;
#124355=CARTESIAN_POINT('Ctrl Pts',(-0.89661686844318,-2.65532131305562,
-0.856729861320318)) ;
#124356=CARTESIAN_POINT('Ctrl Pts',(-1.08716606259604,-2.63354835571964,
-0.59584965946805)) ;
#124357=CARTESIAN_POINT('Ctrl Pts',(-1.15543913531375,-2.62263553183912,
-0.449371440771829)) ;
#124358=CARTESIAN_POINT('Ctrl Pts',(-1.21744939388122,-2.60574934374318,
-0.197523456591343)) ;
#124359=CARTESIAN_POINT('Ctrl Pts',(-1.2293670625,-2.59955296821977,-0.0988512871362581)) ;
#124360=CARTESIAN_POINT('Ctrl Pts',(-1.2293670625,-2.59375000068278,1.57096557984454E-13)) ;
#124361=CARTESIAN_POINT('Ctrl Pts',(-1.2293670625,-2.46875000068278,2.36529545949438E-13)) ;
#124362=CARTESIAN_POINT('Ctrl Pts',(-1.2293670625,-2.47479559615011,-0.102984359233321)) ;
#124363=CARTESIAN_POINT('Ctrl Pts',(-1.21643218951429,-2.48126625543479,
-0.205741562296177)) ;
#124364=CARTESIAN_POINT('Ctrl Pts',(-1.15082544508,-2.49848123688728,-0.461113980896463)) ;
#124365=CARTESIAN_POINT('Ctrl Pts',(-1.08098469341727,-2.50941445151738,
-0.607034448192572)) ;
#124366=CARTESIAN_POINT('Ctrl Pts',(-0.887634325931833,-2.53117173733727,
-0.866030433706927)) ;
#124367=CARTESIAN_POINT('Ctrl Pts',(-0.765113431653198,-2.54177862439221,
-0.975977143603221)) ;
#124368=CARTESIAN_POINT('Ctrl Pts',(-0.490262894597181,-2.56061314703315,
-1.13813085425707)) ;
#124369=CARTESIAN_POINT('Ctrl Pts',(-0.341894108069714,-2.57057451750811,
-1.19115887646372)) ;
#124370=CARTESIAN_POINT('Ctrl Pts',(-0.0272233677377015,-2.59190464948757,
-1.23971771974343)) ;
#124371=CARTESIAN_POINT('Ctrl Pts',(0.136372501981445,-2.60299408693804,
-1.23249648183158)) ;
#124372=CARTESIAN_POINT('Ctrl Pts',(0.449574226570522,-2.62422464086445,
-1.15539865499199)) ;
#124373=CARTESIAN_POINT('Ctrl Pts',(0.596250201571124,-2.63348147569385,
-1.08698585341061)) ;
#124374=CARTESIAN_POINT('Ctrl Pts',(0.85321269201525,-2.6532217913139,-0.899074644355462)) ;
#124375=CARTESIAN_POINT('Ctrl Pts',(0.961557236992823,-2.66376014660443,
-0.782110627233372)) ;
#124376=CARTESIAN_POINT('Ctrl Pts',(1.1313164616044,-2.68558452870488,-0.508351330077954)) ;
#124377=CARTESIAN_POINT('Ctrl Pts',(1.18903054470321,-2.69666780846138,
-0.352873226563285)) ;
#124378=CARTESIAN_POINT('Ctrl Pts',(1.23877047881811,-2.71695593887551,
-0.0359902076201987)) ;
#124379=CARTESIAN_POINT('Ctrl Pts',(1.23329130610041,-2.72576903638811,
0.121832196860172)) ;
#124380=CARTESIAN_POINT('Ctrl Pts',(1.1626648881041,-2.74626724801714,0.430235050214568)) ;
#124381=CARTESIAN_POINT('Ctrl Pts',(1.0969419384568,-2.7571446637695,0.577582419508308)) ;
#124382=CARTESIAN_POINT('Ctrl Pts',(0.910973195462585,-2.77893790350951,
0.841452648906544)) ;
#124383=CARTESIAN_POINT('Ctrl Pts',(0.791476950211163,-2.78963761801788,
0.954726920172135)) ;
#124384=CARTESIAN_POINT('Ctrl Pts',(0.521340775364793,-2.80874201746369,
1.12419971515682)) ;
#124385=CARTESIAN_POINT('Ctrl Pts',(0.374767996714821,-2.81834614259553,
1.18118791847062)) ;
#124386=CARTESIAN_POINT('Ctrl Pts',(0.062323631990983,-2.83952535846024,
1.23839012382985)) ;
#124387=CARTESIAN_POINT('Ctrl Pts',(-0.100941337485042,-2.85059236565282,
1.23584244565613)) ;
#124388=CARTESIAN_POINT('Ctrl Pts',(-0.417071868631584,-2.87202145036841,
1.1677040626515)) ;
#124389=CARTESIAN_POINT('Ctrl Pts',(-0.566798102144141,-2.88155394679947,
1.10281637829345)) ;
#124390=CARTESIAN_POINT('Ctrl Pts',(-0.829267848896132,-2.90111505220184,
0.921137561263793)) ;
#124391=CARTESIAN_POINT('Ctrl Pts',(-0.940373407989954,-2.91155892088745,
0.807377158822231)) ;
#124392=CARTESIAN_POINT('Ctrl Pts',(-1.11696887428682,-2.93329854470353,
0.539008591937846)) ;
#124393=CARTESIAN_POINT('Ctrl Pts',(-1.17875668419664,-2.94439782077258,
0.385609964753008)) ;
#124394=CARTESIAN_POINT('Ctrl Pts',(-1.2224733540385,-2.95969010605744,
0.150351684495328)) ;
#124395=CARTESIAN_POINT('Ctrl Pts',(-1.2293670625,-2.96433685050023,0.0751762909392223)) ;
#124396=CARTESIAN_POINT('Ctrl Pts',(-1.2293670625,-2.96875000068279,-2.42861286636753E-16)) ;
#124397=CARTESIAN_POINT('Origin',(1.38777878078145E-16,-6.28125000068279,
-2.77555756156289E-16)) ;
#124398=CARTESIAN_POINT('',(-1.2293670625,-3.59375000068281,-1.33093873159813E-13)) ;
#124399=CARTESIAN_POINT('',(-1.2293670625,-3.4687500006828,-6.19008217057184E-14)) ;
#124400=CARTESIAN_POINT('',(-1.2293670625,-6.28125000068279,-7.05665556119359E-16)) ;
#124401=CARTESIAN_POINT('Ctrl Pts',(-1.2293670625,-3.59375000068281,-2.6477084413834E-13)) ;
#124402=CARTESIAN_POINT('Ctrl Pts',(-1.22936706250002,-3.58760601015228,
0.104660480732079)) ;
#124403=CARTESIAN_POINT('Ctrl Pts',(-1.21600778734524,-3.58102380425275,
0.209072808136304)) ;
#124404=CARTESIAN_POINT('Ctrl Pts',(-1.14892130661534,-3.56367559742544,
0.465860342851234)) ;
#124405=CARTESIAN_POINT('Ctrl Pts',(-1.07844627114001,-3.55273443320507,
0.611550024384985)) ;
#124406=CARTESIAN_POINT('Ctrl Pts',(-0.883965747763156,-3.53098418698764,
0.869773597210837)) ;
#124407=CARTESIAN_POINT('Ctrl Pts',(-0.760985628392447,-3.52039238066184,
0.979198279041553)) ;
#124408=CARTESIAN_POINT('Ctrl Pts',(-0.485411672162505,-3.50160004833661,
1.14021562787906)) ;
#124409=CARTESIAN_POINT('Ctrl Pts',(-0.336759268855858,-3.49157741591188,
1.19262899043324)) ;
#124410=CARTESIAN_POINT('Ctrl Pts',(-0.0217473940391149,-3.47022415994073,
1.23983515216573)) ;
#124411=CARTESIAN_POINT('Ctrl Pts',(0.141888301312603,-3.45913202288751,
1.231883176924)) ;
#124412=CARTESIAN_POINT('Ctrl Pts',(0.454623961896689,-3.43793306137013,
1.15339476994935)) ;
#124413=CARTESIAN_POINT('Ctrl Pts',(0.60082851666236,-3.42871357231804,
1.08443438350177)) ;
#124414=CARTESIAN_POINT('Ctrl Pts',(0.856923708288166,-3.40894549540734,
0.895549536489281)) ;
#124415=CARTESIAN_POINT('Ctrl Pts',(0.964825898786098,-3.39839291846952,
0.778087865678279)) ;
#124416=CARTESIAN_POINT('Ctrl Pts',(1.13349582868348,-3.37655660776514,
0.503496464814202)) ;
#124417=CARTESIAN_POINT('Ctrl Pts',(1.19056336220522,-3.36547660348108,
0.34770087212176)) ;
#124418=CARTESIAN_POINT('Ctrl Pts',(1.23890533877188,-3.34522346818345,
0.0306068701632447)) ;
#124419=CARTESIAN_POINT('Ctrl Pts',(1.2327486931859,-3.33640267430905,-0.127111222554901)) ;
#124420=CARTESIAN_POINT('Ctrl Pts',(1.16082336244135,-3.31587865740719,
-0.435203731035599)) ;
#124421=CARTESIAN_POINT('Ctrl Pts',(1.09443883629321,-3.30499179111457,
-0.582330125223285)) ;
#124422=CARTESIAN_POINT('Ctrl Pts',(0.910768604013118,-3.28360944903533,
-0.840527919120294)) ;
#124423=CARTESIAN_POINT('Ctrl Pts',(0.796088100862452,-3.2733038140609,
-0.94986956932987)) ;
#124424=CARTESIAN_POINT('Ctrl Pts',(0.52621714509681,-3.25399174662172,
-1.1230330318379)) ;
#124425=CARTESIAN_POINT('Ctrl Pts',(0.372237511017996,-3.243982328383,-1.18303829228058)) ;
#124426=CARTESIAN_POINT('Ctrl Pts',(0.0522678883627475,-3.2222930087041,
-1.23877414166441)) ;
#124427=CARTESIAN_POINT('Ctrl Pts',(-0.110332419279826,-3.21127105598534,
-1.23495833974307)) ;
#124428=CARTESIAN_POINT('Ctrl Pts',(-0.419620068981708,-3.19030581981244,
-1.16598981359416)) ;
#124429=CARTESIAN_POINT('Ctrl Pts',(-0.563793406330703,-3.18108853879862,
-1.10350877964673)) ;
#124430=CARTESIAN_POINT('Ctrl Pts',(-0.827245262968623,-3.1616164357492,
-0.923913104369628)) ;
#124431=CARTESIAN_POINT('Ctrl Pts',(-0.942369880473406,-3.15080100137205,
-0.806143629847639)) ;
#124432=CARTESIAN_POINT('Ctrl Pts',(-1.11784570469313,-3.12898528792528,
-0.535832480147024)) ;
#124433=CARTESIAN_POINT('Ctrl Pts',(-1.17778645929249,-3.11819824637287,
-0.386686248209585)) ;
#124434=CARTESIAN_POINT('Ctrl Pts',(-1.22211804529408,-3.10304610177953,
-0.154170231946575)) ;
#124435=CARTESIAN_POINT('Ctrl Pts',(-1.2293670625,-3.09827547011273,-0.0770896054808835)) ;
#124436=CARTESIAN_POINT('Ctrl Pts',(-1.2293670625,-3.09375000068279,-1.38777878078145E-16)) ;
#124437=CARTESIAN_POINT('Ctrl Pts',(-1.2293670625,-2.96875000068279,-2.42861286636753E-16)) ;
#124438=CARTESIAN_POINT('Ctrl Pts',(-1.2293670625,-2.9735185044223,-0.0812296000898806)) ;
#124439=CARTESIAN_POINT('Ctrl Pts',(-1.22131876533305,-2.97855794949859,
-0.16242789356958)) ;
#124440=CARTESIAN_POINT('Ctrl Pts',(-1.17378991834763,-2.99403993871629,
-0.398716744783189)) ;
#124441=CARTESIAN_POINT('Ctrl Pts',(-1.11225471253075,-3.00485328327833,
-0.54739048138406)) ;
#124442=CARTESIAN_POINT('Ctrl Pts',(-0.933870791753979,-3.02666602419055,
-0.81597200478877)) ;
#124443=CARTESIAN_POINT('Ctrl Pts',(-0.817526375905969,-3.03745123578314,
-0.932522395069542)) ;
#124444=CARTESIAN_POINT('Ctrl Pts',(-0.552222673387235,-3.05682321399114,
-1.10934331903335)) ;
#124445=CARTESIAN_POINT('Ctrl Pts',(-0.407401061733189,-3.06613409204707,
-1.17031584431765)) ;
#124446=CARTESIAN_POINT('Ctrl Pts',(-0.0972396532885814,-3.08715855644462,
-1.23608004546991)) ;
#124447=CARTESIAN_POINT('Ctrl Pts',(0.0655662515812561,-3.09819444568632,
-1.23816371320781)) ;
#124448=CARTESIAN_POINT('Ctrl Pts',(0.384508316336356,-3.11981411177874,
-1.17902676959833)) ;
#124449=CARTESIAN_POINT('Ctrl Pts',(0.537318554711961,-3.12968216870808,
-1.11768136289317)) ;
#124450=CARTESIAN_POINT('Ctrl Pts',(0.805184905728154,-3.14906263877633,
-0.942195329204265)) ;
#124451=CARTESIAN_POINT('Ctrl Pts',(0.918912938143374,-3.15940697617733,
-0.831644489027856)) ;
#124452=CARTESIAN_POINT('Ctrl Pts',(1.1020653917792,-3.18104846412195,-0.568733306817234)) ;
#124453=CARTESIAN_POINT('Ctrl Pts',(1.16778794606958,-3.19215532625225,
-0.417477179767121)) ;
#124454=CARTESIAN_POINT('Ctrl Pts',(1.23513416838476,-3.21287233027657,
-0.10345346149256)) ;
#124455=CARTESIAN_POINT('Ctrl Pts',(1.23820309414711,-3.22172462798742,
0.0557731004087756)) ;
#124456=CARTESIAN_POINT('Ctrl Pts',(1.18290380469142,-3.24220806707491,
0.372773431072468)) ;
#124457=CARTESIAN_POINT('Ctrl Pts',(1.12270956248791,-3.25330205090422,
0.527001953763053)) ;
#124458=CARTESIAN_POINT('Ctrl Pts',(0.948782669306098,-3.2750768270657,
0.797510028537988)) ;
#124459=CARTESIAN_POINT('Ctrl Pts',(0.838751730640217,-3.2855586719991,
0.912537773932019)) ;
#124460=CARTESIAN_POINT('Ctrl Pts',(0.57844541351642,-3.30519078524983,
1.09667523862282)) ;
#124461=CARTESIAN_POINT('Ctrl Pts',(0.429929124653981,-3.31460701471273,
1.16295792032336)) ;
#124462=CARTESIAN_POINT('Ctrl Pts',(0.114942506030843,-3.33595855867868,
1.23464275025172)) ;
#124463=CARTESIAN_POINT('Ctrl Pts',(-0.0484687036745916,-3.34703547884692,
1.23903305836949)) ;
#124464=CARTESIAN_POINT('Ctrl Pts',(-0.361800080875293,-3.36827482134806,
1.18523743760659)) ;
#124465=CARTESIAN_POINT('Ctrl Pts',(-0.509077341519926,-3.37801258291071,
1.12981703328546)) ;
#124466=CARTESIAN_POINT('Ctrl Pts',(-0.781090789954048,-3.39701056694208,
0.963240827763799)) ;
#124467=CARTESIAN_POINT('Ctrl Pts',(-0.901797856044311,-3.40767444388521,
0.851276103172143)) ;
#124468=CARTESIAN_POINT('Ctrl Pts',(-1.0907089679849,-3.42945540836165,
0.589313755601145)) ;
#124469=CARTESIAN_POINT('Ctrl Pts',(-1.15806817539359,-3.4403558606355,
0.442518662013712)) ;
#124470=CARTESIAN_POINT('Ctrl Pts',(-1.21802169125973,-3.45705071436777,
0.192742523089721)) ;
#124471=CARTESIAN_POINT('Ctrl Pts',(-1.22936706250001,-3.46308811210588,
0.0964480621133391)) ;
#124472=CARTESIAN_POINT('Ctrl Pts',(-1.2293670625,-3.4687500006828,-1.23095977855318E-13)) ;
#124473=CARTESIAN_POINT('Origin',(1.38777878078145E-16,-6.28125000068279,
-2.77555756156289E-16)) ;
#124474=CARTESIAN_POINT('',(-1.2293670625,-4.09375000068281,-1.69945164818064E-13)) ;
#124475=CARTESIAN_POINT('',(-1.2293670625,-3.96875000068281,-1.99426391777733E-13)) ;
#124476=CARTESIAN_POINT('',(-1.2293670625,-6.28125000068279,-7.05665556119359E-16)) ;
#124477=CARTESIAN_POINT('Ctrl Pts',(-1.2293670625,-4.09375000068281,-3.38930272736349E-13)) ;
#124478=CARTESIAN_POINT('Ctrl Pts',(-1.22936706250003,-4.08638052380908,
0.125536162289958)) ;
#124479=CARTESIAN_POINT('Ctrl Pts',(-1.21014633715312,-4.07839389712964,
0.250488139698543)) ;
#124480=CARTESIAN_POINT('Ctrl Pts',(-1.12362683665224,-4.05939449681373,
0.524183451846886)) ;
#124481=CARTESIAN_POINT('Ctrl Pts',(-1.0453277057579,-4.04836981458519,
0.666778586456919)) ;
#124482=CARTESIAN_POINT('Ctrl Pts',(-0.836612973503375,-4.02669358615773,
0.915523170792202)) ;
#124483=CARTESIAN_POINT('Ctrl Pts',(-0.707547991574335,-4.01671153668759,
1.01855193211573)) ;
#124484=CARTESIAN_POINT('Ctrl Pts',(-0.422457351582659,-3.99738650833981,
1.16513818239883)) ;
#124485=CARTESIAN_POINT('Ctrl Pts',(-0.270315676817875,-3.98707349989521,
1.20951433049297)) ;
#124486=CARTESIAN_POINT('Ctrl Pts',(0.0484689556015864,-3.96546450544165,
1.23919865340816)) ;
#124487=CARTESIAN_POINT('Ctrl Pts',(0.212332360409137,-3.95435693297571,
1.22183753073967)) ;
#124488=CARTESIAN_POINT('Ctrl Pts',(0.518875100939212,-3.93357776200495,
1.12565795121915)) ;
#124489=CARTESIAN_POINT('Ctrl Pts',(0.659137378893126,-3.92469835485736,
1.0497013584745)) ;
#124490=CARTESIAN_POINT('Ctrl Pts',(0.903890852904691,-3.90457848394732,
0.848275694268292)) ;
#124491=CARTESIAN_POINT('Ctrl Pts',(1.00583041356504,-3.89385659734632,
0.724487373483557)) ;
#124492=CARTESIAN_POINT('Ctrl Pts',(1.15895567003433,-3.87204333499161,
0.441313870872362)) ;
#124493=CARTESIAN_POINT('Ctrl Pts',(1.20722606073727,-3.86116254905237,
0.283832852155816)) ;
#124494=CARTESIAN_POINT('Ctrl Pts',(1.23874930343796,-3.84146129761652,
-0.0335703241386011)) ;
#124495=CARTESIAN_POINT('Ctrl Pts',(1.2245344497137,-3.8324241078749,-0.190142053275185)) ;
#124496=CARTESIAN_POINT('Ctrl Pts',(1.13699604646107,-3.81159718918911,
-0.494380163809215)) ;
#124497=CARTESIAN_POINT('Ctrl Pts',(1.06270206926562,-3.8006118661332,-0.638617206841338)) ;
#124498=CARTESIAN_POINT('Ctrl Pts',(0.861339561302336,-3.7789000006111,
-0.892213663848438)) ;
#124499=CARTESIAN_POINT('Ctrl Pts',(0.73554048225724,-3.76860902331144,
-0.998440434382698)) ;
#124500=CARTESIAN_POINT('Ctrl Pts',(0.455535097815912,-3.74962870185291,
-1.15254829981474)) ;
#124501=CARTESIAN_POINT('Ctrl Pts',(0.305162198330013,-3.73943559082904,
-1.20113795706868)) ;
#124502=CARTESIAN_POINT('Ctrl Pts',(-0.0116982000569486,-3.71795703165468,
-1.24002767785997)) ;
#124503=CARTESIAN_POINT('Ctrl Pts',(-0.17550792565351,-3.70685309786405,
-1.22760302835133)) ;
#124504=CARTESIAN_POINT('Ctrl Pts',(-0.485343860960918,-3.68585069584499,
-1.14065819846299)) ;
#124505=CARTESIAN_POINT('Ctrl Pts',(-0.628694615511167,-3.67682560507665,
-1.06836209807631)) ;
#124506=CARTESIAN_POINT('Ctrl Pts',(-0.879440832705246,-3.65688903408383,
-0.873518788308913)) ;
#124507=CARTESIAN_POINT('Ctrl Pts',(-0.984571189267261,-3.64625273681576,
-0.753030655278479)) ;
#124508=CARTESIAN_POINT('Ctrl Pts',(-1.14645061853887,-3.62435139506056,
-0.473410978480525)) ;
#124509=CARTESIAN_POINT('Ctrl Pts',(-1.19950278771445,-3.6132961104085,
-0.315718203385222)) ;
#124510=CARTESIAN_POINT('Ctrl Pts',(-1.22621928597872,-3.59982319482307,
-0.101637122233833)) ;
#124511=CARTESIAN_POINT('Ctrl Pts',(-1.22936706249999,-3.59673190874796,
-0.0507956400729371)) ;
#124512=CARTESIAN_POINT('Ctrl Pts',(-1.2293670625,-3.59375000068281,-2.65482080763506E-13)) ;
#124513=CARTESIAN_POINT('Ctrl Pts',(-1.2293670625,-3.4687500006828,-1.23095977855318E-13)) ;
#124514=CARTESIAN_POINT('Ctrl Pts',(-1.22936706249999,-3.47222775039935,
-0.0592421090809118)) ;
#124515=CARTESIAN_POINT('Ctrl Pts',(-1.2250856159725,-3.47585300320359,
-0.118524981385997)) ;
#124516=CARTESIAN_POINT('Ctrl Pts',(-1.19277723758023,-3.48995421553719,
-0.340080378925659)) ;
#124517=CARTESIAN_POINT('Ctrl Pts',(-1.13666371204228,-3.50102902580151,
-0.496338290285139)) ;
#124518=CARTESIAN_POINT('Ctrl Pts',(-0.969603180734232,-3.52288219124833,
-0.772145991817219)) ;
#124519=CARTESIAN_POINT('Ctrl Pts',(-0.862355731305695,-3.5334553732651,
-0.890336677038728)) ;
#124520=CARTESIAN_POINT('Ctrl Pts',(-0.6075371086556,-3.55326408644235,
-1.08065077443381)) ;
#124521=CARTESIAN_POINT('Ctrl Pts',(-0.462022010915018,-3.56243158048319,
-1.15041362155065)) ;
#124522=CARTESIAN_POINT('Ctrl Pts',(-0.149974532350621,-3.5835838931978,
-1.23093887072348)) ;
#124523=CARTESIAN_POINT('Ctrl Pts',(0.0137138229336498,-3.59467959983398,
-1.23996367402928)) ;
#124524=CARTESIAN_POINT('Ctrl Pts',(0.329092262799837,-3.61605770362185,
-1.19476309977395)) ;
#124525=CARTESIAN_POINT('Ctrl Pts',(0.478175266376449,-3.62616337833069,
-1.14329942778789)) ;
#124526=CARTESIAN_POINT('Ctrl Pts',(0.754804709660387,-3.6449148597313,
-0.98394691504196)) ;
#124527=CARTESIAN_POINT('Ctrl Pts',(0.878493111818562,-3.65547281413675,
-0.875325006304689)) ;
#124528=CARTESIAN_POINT('Ctrl Pts',(1.07470347427421,-3.67722138650442,
-0.618128669913968)) ;
#124529=CARTESIAN_POINT('Ctrl Pts',(1.14610401386665,-3.68817383765985,
-0.472781059897794)) ;
#124530=CARTESIAN_POINT('Ctrl Pts',(1.22791026291866,-3.70889112795589,
-0.167100965425369)) ;
#124531=CARTESIAN_POINT('Ctrl Pts',(1.23918350911488,-3.71782254272044,
-0.0101313563127505)) ;
#124532=CARTESIAN_POINT('Ctrl Pts',(1.20159883077571,-3.73770092954693,
0.306789680728972)) ;
#124533=CARTESIAN_POINT('Ctrl Pts',(1.15033099587973,-3.74862842966255,
0.463335881996003)) ;
#124534=CARTESIAN_POINT('Ctrl Pts',(0.991965571920356,-3.77043063170934,
0.743295564467743)) ;
#124535=CARTESIAN_POINT('Ctrl Pts',(0.887919578162098,-3.78109726087565,
0.864926446702843)) ;
#124536=CARTESIAN_POINT('Ctrl Pts',(0.639228485315649,-3.80109733796104,
1.06203808456671)) ;
#124537=CARTESIAN_POINT('Ctrl Pts',(0.496949753192357,-3.81006398395441,
1.13559806310939)) ;
#124538=CARTESIAN_POINT('Ctrl Pts',(0.188238382595696,-3.83099015672611,
1.22573793466198)) ;
#124539=CARTESIAN_POINT('Ctrl Pts',(0.0243937945375404,-3.84209645368818,
1.23986468914897)) ;
#124540=CARTESIAN_POINT('Ctrl Pts',(-0.293160443086161,-3.86362204514294,
1.20414337576111)) ;
#124541=CARTESIAN_POINT('Ctrl Pts',(-0.444157114198976,-3.87385743887512,
1.15700113913959)) ;
#124542=CARTESIAN_POINT('Ctrl Pts',(-0.72725774007465,-3.89304757300398,
1.00476258948857)) ;
#124543=CARTESIAN_POINT('Ctrl Pts',(-0.855187517823339,-3.90332747876962,
0.898414466008073)) ;
#124544=CARTESIAN_POINT('Ctrl Pts',(-1.05908987483039,-3.92513750554639,
0.644612252868314)) ;
#124545=CARTESIAN_POINT('Ctrl Pts',(-1.13423370611862,-3.93613178141959,
0.500713365577207)) ;
#124546=CARTESIAN_POINT('Ctrl Pts',(-1.2126517599951,-3.95446371636377,
0.233710693139845)) ;
#124547=CARTESIAN_POINT('Ctrl Pts',(-1.22936706250004,-3.96187746419692,
0.117070976735388)) ;
#124548=CARTESIAN_POINT('Ctrl Pts',(-1.2293670625,-3.96875000068281,-3.97772093041482E-13)) ;
#124549=CARTESIAN_POINT('Origin',(1.38777878078145E-16,-6.28125000068279,
-2.77555756156289E-16)) ;
#124550=CARTESIAN_POINT('',(-1.2293670625,-4.59375000068279,-2.88487871326898E-15)) ;
#124551=CARTESIAN_POINT('',(-1.2293670625,-4.46875000068279,-4.21931813261631E-14)) ;
#124552=CARTESIAN_POINT('',(-1.2293670625,-6.28125000068279,-7.05665556119359E-16)) ;
#124553=CARTESIAN_POINT('Ctrl Pts',(-1.2293670625,-4.59375000068279,-5.51642065360625E-15)) ;
#124554=CARTESIAN_POINT('Ctrl Pts',(-1.2293670625,-4.58502896270038,0.148559478272167)) ;
#124555=CARTESIAN_POINT('Ctrl Pts',(-1.20244149704241,-4.57546057872006,
0.29600768244092)) ;
#124556=CARTESIAN_POINT('Ctrl Pts',(-1.09241263142596,-4.55466592437684,
0.586711307991789)) ;
#124557=CARTESIAN_POINT('Ctrl Pts',(-1.00566097257559,-4.54358248897905,
0.725427210618369)) ;
#124558=CARTESIAN_POINT('Ctrl Pts',(-0.784228883049274,-4.52228968246801,
0.960297982609938)) ;
#124559=CARTESIAN_POINT('Ctrl Pts',(-0.652117065633409,-4.51295412039647,
1.05447525637748)) ;
#124560=CARTESIAN_POINT('Ctrl Pts',(-0.361715619769164,-4.4932690961048,
1.18550797902303)) ;
#124561=CARTESIAN_POINT('Ctrl Pts',(-0.20667242902016,-4.48275940677778,
1.22210291679461)) ;
#124562=CARTESIAN_POINT('Ctrl Pts',(0.114924739347508,-4.46095976300325,
1.23492670753276)) ;
#124563=CARTESIAN_POINT('Ctrl Pts',(0.278516439940176,-4.44987060815935,
1.20859199982724)) ;
#124564=CARTESIAN_POINT('Ctrl Pts',(0.578830914555416,-4.42951362367414,
1.09583492247798)) ;
#124565=CARTESIAN_POINT('Ctrl Pts',(0.713621918901493,-4.42071100408087,
1.01323505807178)) ;
#124566=CARTESIAN_POINT('Ctrl Pts',(0.947202221169259,-4.40026400633689,
0.799786082210475)) ;
#124567=CARTESIAN_POINT('Ctrl Pts',(1.04297114101472,-4.38940580677613,
0.670113102222645)) ;
#124568=CARTESIAN_POINT('Ctrl Pts',(1.18098138091927,-4.36760464824602,
0.378419124657103)) ;
#124569=CARTESIAN_POINT('Ctrl Pts',(1.22071531321839,-4.35687728656373,
0.218623101719924)) ;
#124570=CARTESIAN_POINT('Ctrl Pts',(1.23516206743971,-4.33768862691041,
-0.0999073888403545)) ;
#124571=CARTESIAN_POINT('Ctrl Pts',(1.212586789702,-4.32818351361548,-0.255480936687184)) ;
#124572=CARTESIAN_POINT('Ctrl Pts',(1.10859373622348,-4.30705247791321,
-0.555399465164944)) ;
#124573=CARTESIAN_POINT('Ctrl Pts',(1.02608340058017,-4.29599431067272,
-0.696133663689217)) ;
#124574=CARTESIAN_POINT('Ctrl Pts',(0.811004123444689,-4.27450452743128,
-0.93802765534849)) ;
#124575=CARTESIAN_POINT('Ctrl Pts',(0.68042538038046,-4.264873015331,-1.03664089660206)) ;
#124576=CARTESIAN_POINT('Ctrl Pts',(0.392686325852142,-4.24536846272385,
-1.17555839978656)) ;
#124577=CARTESIAN_POINT('Ctrl Pts',(0.239067393119562,-4.23495531752239,
-1.21612778762906)) ;
#124578=CARTESIAN_POINT('Ctrl Pts',(-0.0812104726257985,-4.21324510341337,
-1.23754148401705)) ;
#124579=CARTESIAN_POINT('Ctrl Pts',(-0.244999659907664,-4.20214256182388,
-1.21576769693668)) ;
#124580=CARTESIAN_POINT('Ctrl Pts',(-0.548516914349574,-4.18156847511833,
-1.11140752058824)) ;
#124581=CARTESIAN_POINT('Ctrl Pts',(-0.686070105373153,-4.17275723050083,
-1.03218467955117)) ;
#124582=CARTESIAN_POINT('Ctrl Pts',(-0.925376763970217,-4.15247569306073,
-0.824860368756792)) ;
#124583=CARTESIAN_POINT('Ctrl Pts',(-1.02434314788367,-4.14168358188332,
-0.698159235325802)) ;
#124584=CARTESIAN_POINT('Ctrl Pts',(-1.17014351158204,-4.11986824510788,
-0.410721366954031)) ;
#124585=CARTESIAN_POINT('Ctrl Pts',(-1.21425721494069,-4.10905844566451,
-0.25204971093212)) ;
#124586=CARTESIAN_POINT('Ctrl Pts',(-1.22828505133293,-4.0972847201261,
-0.0595878667026296)) ;
#124587=CARTESIAN_POINT('Ctrl Pts',(-1.22936706249999,-4.09549818489378,
-0.0297796357305136)) ;
#124588=CARTESIAN_POINT('Ctrl Pts',(-1.2293670625,-4.09375000068281,-3.3918466408001E-13)) ;
#124589=CARTESIAN_POINT('Ctrl Pts',(-1.2293670625,-3.96875000068281,-3.98147117999346E-13)) ;
#124590=CARTESIAN_POINT('Ctrl Pts',(-1.22936706249999,-3.97099398318985,
-0.0382253661975134)) ;
#124591=CARTESIAN_POINT('Ctrl Pts',(-1.22758434631669,-3.9733006693718,
-0.0764896133558483)) ;
#124592=CARTESIAN_POINT('Ctrl Pts',(-1.20879117961218,-3.98571363210003,
-0.277089348885761)) ;
#124593=CARTESIAN_POINT('Ctrl Pts',(-1.16140207282899,-3.99657996572339,
-0.434832987550155)) ;
#124594=CARTESIAN_POINT('Ctrl Pts',(-1.00982419566573,-4.01839494669545,
-0.718929145995987)) ;
#124595=CARTESIAN_POINT('Ctrl Pts',(-0.908509961324784,-4.02913233953647,
-0.843342641846237)) ;
#124596=CARTESIAN_POINT('Ctrl Pts',(-0.664912394162676,-4.04928690955548,
-1.04602675496179)) ;
#124597=CARTESIAN_POINT('Ctrl Pts',(-0.525232762040495,-4.05814680439437,
-1.12268103208231)) ;
#124598=CARTESIAN_POINT('Ctrl Pts',(-0.219329781308588,-4.07888260888969,
-1.22061340271302)) ;
#124599=CARTESIAN_POINT('Ctrl Pts',(-0.0554725601817823,-4.08998976219138,
-1.23891705515827)) ;
#124600=CARTESIAN_POINT('Ctrl Pts',(0.263648966044517,-4.1116215931799,
-1.21099598897818)) ;
#124601=CARTESIAN_POINT('Ctrl Pts',(0.416114393967901,-4.12195654741327,
-1.16742976198749)) ;
#124602=CARTESIAN_POINT('Ctrl Pts',(0.701777012591598,-4.14132034765226,
-1.0224853899473)) ;
#124603=CARTESIAN_POINT('Ctrl Pts',(0.831168411807016,-4.15122215030892,
-0.920410477317314)) ;
#124604=CARTESIAN_POINT('Ctrl Pts',(1.04126155347177,-4.1728589190223,-0.673133898854699)) ;
#124605=CARTESIAN_POINT('Ctrl Pts',(1.12046919701639,-4.18389151887796,
-0.530928420580006)) ;
#124606=CARTESIAN_POINT('Ctrl Pts',(1.21781227475221,-4.20490157974945,
-0.229231285843895)) ;
#124607=CARTESIAN_POINT('Ctrl Pts',(1.23702161082716,-4.214188766796,-0.0732794835073471)) ;
#124608=CARTESIAN_POINT('Ctrl Pts',(1.21573099869258,-4.23358520739107,
0.244839171091622)) ;
#124609=CARTESIAN_POINT('Ctrl Pts',(1.172561374576,-4.2443778941776,0.403764384087774)) ;
#124610=CARTESIAN_POINT('Ctrl Pts',(1.02843398404133,-4.26619158332599,
0.692140077282357)) ;
#124611=CARTESIAN_POINT('Ctrl Pts',(0.930151239543393,-4.27699862077546,
0.819490173332727)) ;
#124612=CARTESIAN_POINT('Ctrl Pts',(0.692079448142443,-4.29731625571283,
1.02814234181259)) ;
#124613=CARTESIAN_POINT('Ctrl Pts',(0.555129934481888,-4.30612020785312,
1.10809793093287)) ;
#124614=CARTESIAN_POINT('Ctrl Pts',(0.252301527439119,-4.32664760065277,
1.21428676574491)) ;
#124615=CARTESIAN_POINT('Ctrl Pts',(0.0885448104424789,-4.33774794122583,
1.23705126113019)) ;
#124616=CARTESIAN_POINT('Ctrl Pts',(-0.232038974862563,-4.35947889226316,
1.21749986572218)) ;
#124617=CARTESIAN_POINT('Ctrl Pts',(-0.38597614135646,-4.36991360911797,
1.17779036275969)) ;
#124618=CARTESIAN_POINT('Ctrl Pts',(-0.674299787885864,-4.3894577886206,
1.0405887745593)) ;
#124619=CARTESIAN_POINT('Ctrl Pts',(-0.805213866067154,-4.39901932993295,
0.942949798707443)) ;
#124620=CARTESIAN_POINT('Ctrl Pts',(-1.02169191086748,-4.4204666797767,
0.702586222304148)) ;
#124621=CARTESIAN_POINT('Ctrl Pts',(-1.10513306619431,-4.43153112845838,
0.562282430875642)) ;
#124622=CARTESIAN_POINT('Ctrl Pts',(-1.20563624208665,-4.45162168231164,
0.278073222839467)) ;
#124623=CARTESIAN_POINT('Ctrl Pts',(-1.22936706250001,-4.46056203071758,
0.139478872651708)) ;
#124624=CARTESIAN_POINT('Ctrl Pts',(-1.2293670625,-4.4687500006828,-8.41687830543947E-14)) ;
#124625=CARTESIAN_POINT('Origin',(1.38777878078145E-16,-6.28125000068279,
-2.77555756156289E-16)) ;
#124626=CARTESIAN_POINT('',(-1.2293670625,-5.09375000068279,4.13369617262378E-14)) ;
#124627=CARTESIAN_POINT('',(-1.2293670625,-4.96875000068279,8.00274656689887E-16)) ;
#124628=CARTESIAN_POINT('',(-1.2293670625,-6.28125000068279,-7.05665556119359E-16)) ;
#124629=CARTESIAN_POINT('Ctrl Pts',(-1.2293670625,-5.09375000068279,8.3379589008595E-14)) ;
#124630=CARTESIAN_POINT('Ctrl Pts',(-1.2293670625,-5.09284878208426,0.0153519070867942)) ;
#124631=CARTESIAN_POINT('Ctrl Pts',(-1.22907950061357,-5.09193720633504,
0.0307142202611759)) ;
#124632=CARTESIAN_POINT('Ctrl Pts',(-1.22262209133582,-5.08161187395681,
0.202874040436789)) ;
#124633=CARTESIAN_POINT('Ctrl Pts',(-1.18677932781036,-5.07134546323376,
0.357064511027953)) ;
#124634=CARTESIAN_POINT('Ctrl Pts',(-1.05663006087162,-5.04978606774068,
0.649178684474244)) ;
#124635=CARTESIAN_POINT('Ctrl Pts',(-0.961362253967709,-5.03867876569656,
0.78338434573489)) ;
#124636=CARTESIAN_POINT('Ctrl Pts',(-0.727302402490689,-5.01781019475081,
1.00373778868626)) ;
#124637=CARTESIAN_POINT('Ctrl Pts',(-0.592038632639754,-5.00888167024263,
1.0890111704998)) ;
#124638=CARTESIAN_POINT('Ctrl Pts',(-0.296290879588158,-4.98883424353062,
1.20363887658012)) ;
#124639=CARTESIAN_POINT('Ctrl Pts',(-0.138605626097923,-4.97814546050423,
1.23179093614033)) ;
#124640=CARTESIAN_POINT('Ctrl Pts',(0.183107568848696,-4.95633795180321,
1.22654437988664)) ;
#124641=CARTESIAN_POINT('Ctrl Pts',(0.344050664648374,-4.9454283341153,
1.19146438075983)) ;
#124642=CARTESIAN_POINT('Ctrl Pts',(0.636281586836292,-4.92561929774868,
1.06339132794893)) ;
#124643=CARTESIAN_POINT('Ctrl Pts',(0.765869002702726,-4.91665000809934,
0.97422244440075)) ;
#124644=CARTESIAN_POINT('Ctrl Pts',(0.988082378871063,-4.8958895101667,
0.748870417339189)) ;
#124645=CARTESIAN_POINT('Ctrl Pts',(1.07731754330718,-4.88492371284935,
0.613592286118149)) ;
#124646=CARTESIAN_POINT('Ctrl Pts',(1.19972527392039,-4.8631886143498,0.3140155024508)) ;
#124647=CARTESIAN_POINT('Ctrl Pts',(1.23072524817926,-4.85273861333006,
0.152333359387764)) ;
#124648=CARTESIAN_POINT('Ctrl Pts',(1.22797339605001,-4.83389663328735,
-0.167043634183287)) ;
#124649=CARTESIAN_POINT('Ctrl Pts',(1.19677229142187,-4.82375624256793,
-0.321767266211094)) ;
#124650=CARTESIAN_POINT('Ctrl Pts',(1.07579219170482,-4.80233776217868,
-0.616774827025522)) ;
#124651=CARTESIAN_POINT('Ctrl Pts',(0.984951348674464,-4.7912382756839,
-0.75340326223757)) ;
#124652=CARTESIAN_POINT('Ctrl Pts',(0.757438346836806,-4.77014429628392,
-0.981376275633077)) ;
#124653=CARTESIAN_POINT('Ctrl Pts',(0.623829483135525,-4.76103663080903,
-1.07128051838844)) ;
#124654=CARTESIAN_POINT('Ctrl Pts',(0.330862225988127,-4.74117768156569,
-1.19453918189261)) ;
#124655=CARTESIAN_POINT('Ctrl Pts',(0.174511857316672,-4.73057938445271,
-1.22716045151316)) ;
#124656=CARTESIAN_POINT('Ctrl Pts',(-0.148167291193781,-4.70870639804956,
-1.23144051771096)) ;
#124657=CARTESIAN_POINT('Ctrl Pts',(-0.311442806770412,-4.69763867598367,
-1.20059131312558)) ;
#124658=CARTESIAN_POINT('Ctrl Pts',(-0.608505635138163,-4.67750210615645,
-1.07957038658589)) ;
#124659=CARTESIAN_POINT('Ctrl Pts',(-0.740605368455963,-4.66864436882701,
-0.993609634978932)) ;
#124660=CARTESIAN_POINT('Ctrl Pts',(-0.96840469503832,-4.64803545715341,
-0.774064870652292)) ;
#124661=CARTESIAN_POINT('Ctrl Pts',(-1.06087962465526,-4.63711863061326,
-0.641491416807209)) ;
#124662=CARTESIAN_POINT('Ctrl Pts',(-1.19095276777593,-4.61534849633566,
-0.345743440309638)) ;
#124663=CARTESIAN_POINT('Ctrl Pts',(-1.22626597007615,-4.60471213040813,
-0.184945184885094)) ;
#124664=CARTESIAN_POINT('Ctrl Pts',(-1.22930203210093,-4.59460948656494,
-0.0146034612325995)) ;
#124665=CARTESIAN_POINT('Ctrl Pts',(-1.2293670625,-4.59417857029751,-0.00730051611917697)) ;
#124666=CARTESIAN_POINT('Ctrl Pts',(-1.2293670625,-4.59375000068279,-5.06409187041859E-15)) ;
#124667=CARTESIAN_POINT('Ctrl Pts',(-1.2293670625,-4.46875000068279,-8.36806970962069E-14)) ;
#124668=CARTESIAN_POINT('Ctrl Pts',(-1.2293670625,-4.46969418767222,-0.0160838568556484)) ;
#124669=CARTESIAN_POINT('Ctrl Pts',(-1.22905142635401,-4.47064969040176,
-0.032178240313783)) ;
#124670=CARTESIAN_POINT('Ctrl Pts',(-1.22201498643679,-4.48139941711593,
-0.211233148868625)) ;
#124671=CARTESIAN_POINT('Ctrl Pts',(-1.18325041985583,-4.4921074897812,
-0.371260254487391)) ;
#124672=CARTESIAN_POINT('Ctrl Pts',(-1.04697425945045,-4.51390327251257,
-0.663863828685305)) ;
#124673=CARTESIAN_POINT('Ctrl Pts',(-0.951921929457506,-4.52477501772297,
-0.794181276872157)) ;
#124674=CARTESIAN_POINT('Ctrl Pts',(-0.719608812587659,-4.54525794704699,
-1.00897394300623)) ;
#124675=CARTESIAN_POINT('Ctrl Pts',(-0.585415954352627,-4.55406725307158,
-1.09231439546215)) ;
#124676=CARTESIAN_POINT('Ctrl Pts',(-0.285812911339319,-4.57437601276808,
-1.2069010047664)) ;
#124677=CARTESIAN_POINT('Ctrl Pts',(-0.122280738326348,-4.58546113250172,
-1.23423319108302)) ;
#124678=CARTESIAN_POINT('Ctrl Pts',(0.199574657571679,-4.6072782803737,
-1.22329361058302)) ;
#124679=CARTESIAN_POINT('Ctrl Pts',(0.354915451505969,-4.61780814289895,
-1.18757326266864)) ;
#124680=CARTESIAN_POINT('Ctrl Pts',(0.645889580423866,-4.63753198683143,
-1.05826043376743)) ;
#124681=CARTESIAN_POINT('Ctrl Pts',(0.77833354374751,-4.64681167308246,
-0.965037010195778)) ;
#124682=CARTESIAN_POINT('Ctrl Pts',(1.00112632899522,-4.66806086570081,
-0.731694781884955)) ;
#124683=CARTESIAN_POINT('Ctrl Pts',(1.08879073817631,-4.67914860187923,
-0.593432593788058)) ;
#124684=CARTESIAN_POINT('Ctrl Pts',(1.20327793618126,-4.70046498019187,
-0.296415623447903)) ;
#124685=CARTESIAN_POINT('Ctrl Pts',(1.23113924151489,-4.71039075322585,
-0.141373349843462)) ;
#124686=CARTESIAN_POINT('Ctrl Pts',(1.2273366077552,-4.72925026045624,0.177695543471893)) ;
#124687=CARTESIAN_POINT('Ctrl Pts',(1.1929760443945,-4.73986600719604,0.338692565429254)) ;
#124688=CARTESIAN_POINT('Ctrl Pts',(1.06462297287925,-4.76162728401739,
0.635282742420915)) ;
#124689=CARTESIAN_POINT('Ctrl Pts',(0.972866586397243,-4.77255569380347,
0.768468363411924)) ;
#124690=CARTESIAN_POINT('Ctrl Pts',(0.746314148313346,-4.79319885597278,
0.989316462975599)) ;
#124691=CARTESIAN_POINT('Ctrl Pts',(0.614782536371606,-4.80207662289861,
1.07599647139047)) ;
#124692=CARTESIAN_POINT('Ctrl Pts',(0.318422776110228,-4.82216553486134,
1.19877238766902)) ;
#124693=CARTESIAN_POINT('Ctrl Pts',(0.155230107174869,-4.83322764112137,
1.23058301764731)) ;
#124694=CARTESIAN_POINT('Ctrl Pts',(-0.167650703191224,-4.85511429728609,
1.22812774481372)) ;
#124695=CARTESIAN_POINT('Ctrl Pts',(-0.324266271721261,-4.86573057111969,
1.19635781101463)) ;
#124696=CARTESIAN_POINT('Ctrl Pts',(-0.6177715031012,-4.88562598724701,
1.07475189497485)) ;
#124697=CARTESIAN_POINT('Ctrl Pts',(-0.751697555684333,-4.89469335132708,
0.985743499654557)) ;
#124698=CARTESIAN_POINT('Ctrl Pts',(-0.980480609085495,-4.91574452589831,
0.759232914422474)) ;
#124699=CARTESIAN_POINT('Ctrl Pts',(-1.07217853127028,-4.92684631372623,
0.623060111779056)) ;
#124700=CARTESIAN_POINT('Ctrl Pts',(-1.1949290402703,-4.94829337115356,
0.328587898550516)) ;
#124701=CARTESIAN_POINT('Ctrl Pts',(-1.22702424319334,-4.95845867067516,
0.173956162690442)) ;
#124702=CARTESIAN_POINT('Ctrl Pts',(-1.22932590429998,-4.96806660773399,
0.0116175694612323)) ;
#124703=CARTESIAN_POINT('Ctrl Pts',(-1.2293670625,-4.96840905022387,0.00580795799728944)) ;
#124704=CARTESIAN_POINT('Ctrl Pts',(-1.2293670625,-4.96875000068279,2.30621486949913E-15)) ;
#124705=CARTESIAN_POINT('Origin',(1.38777878078145E-16,-6.28125000068279,
-2.77555756156289E-16)) ;
#124706=CARTESIAN_POINT('',(-1.2293670625,-5.59375000068276,2.30508168050804E-13)) ;
#124707=CARTESIAN_POINT('',(-1.2293670625,-5.46875000068277,1.7277409858811E-13)) ;
#124708=CARTESIAN_POINT('',(-1.2293670625,-6.28125000068279,-7.05665556119359E-16)) ;
#124709=CARTESIAN_POINT('Ctrl Pts',(-1.2293670625,-5.59375000068276,4.61722001657727E-13)) ;
#124710=CARTESIAN_POINT('Ctrl Pts',(-1.2293670625,-5.59164548201965,0.0358496540482043)) ;
#124711=CARTESIAN_POINT('Ctrl Pts',(-1.22779903349981,-5.5894855426238,
0.071738076682763)) ;
#124712=CARTESIAN_POINT('Ctrl Pts',(-1.21085554071052,-5.57758691020917,
0.264644305792692)) ;
#124713=CARTESIAN_POINT('Ctrl Pts',(-1.16696861853625,-5.56712153675488,
0.417579731695604)) ;
#124714=CARTESIAN_POINT('Ctrl Pts',(-1.02105739078779,-5.54536183800115,
0.704005820693454)) ;
#124715=CARTESIAN_POINT('Ctrl Pts',(-0.918250213710935,-5.53426538160571,
0.833673873163033)) ;
#124716=CARTESIAN_POINT('Ctrl Pts',(-0.673086072626478,-5.51380607448702,
1.04064460195925)) ;
#124717=CARTESIAN_POINT('Ctrl Pts',(-0.534883633508067,-5.50500738668682,
1.1179832669468)) ;
#124718=CARTESIAN_POINT('Ctrl Pts',(-0.234380415239824,-5.48463760810762,
1.21731386882016)) ;
#124719=CARTESIAN_POINT('Ctrl Pts',(-0.0746398841095792,-5.47380950693786,
1.2374189512917)) ;
#124720=CARTESIAN_POINT('Ctrl Pts',(0.247108611652305,-5.45199960535135,
1.2152613505116)) ;
#124721=CARTESIAN_POINT('Ctrl Pts',(0.405949532666192,-5.44123248475606,
1.17181512506259)) ;
#124722=CARTESIAN_POINT('Ctrl Pts',(0.69087078452292,-5.42191893847767,
1.02873323211164)) ;
#124723=CARTESIAN_POINT('Ctrl Pts',(0.815517005212891,-5.41254933387899,
0.933033347134467)) ;
#124724=CARTESIAN_POINT('Ctrl Pts',(1.02618449411922,-5.39149063919752,
0.695935633721784)) ;
#124725=CARTESIAN_POINT('Ctrl Pts',(1.10857205809211,-5.38044719452686,
0.555381346171666)) ;
#124726=CARTESIAN_POINT('Ctrl Pts',(1.21481446902847,-5.35886860071852,
0.249137507169526)) ;
#124727=CARTESIAN_POINT('Ctrl Pts',(1.23707969576023,-5.34907907533427,
0.0863258158992063)) ;
#124728=CARTESIAN_POINT('Ctrl Pts',(1.21727824541617,-5.32965889532013,
-0.233056998398954)) ;
#124729=CARTESIAN_POINT('Ctrl Pts',(1.17751154204835,-5.31929233582844,
-0.386687976452286)) ;
#124730=CARTESIAN_POINT('Ctrl Pts',(1.03965314901271,-5.29762824188659,
-0.676134781082961)) ;
#124731=CARTESIAN_POINT('Ctrl Pts',(0.940686524261572,-5.28652234596215,
-0.808180976163961)) ;
#124732=CARTESIAN_POINT('Ctrl Pts',(0.701175784845335,-5.265850506202,-1.0220361085325)) ;
#124733=CARTESIAN_POINT('Ctrl Pts',(0.564491191556748,-5.25701435155461,
-1.10342827247686)) ;
#124734=CARTESIAN_POINT('Ctrl Pts',(0.266415312056727,-5.23680911149027,
-1.2106525210943)) ;
#124735=CARTESIAN_POINT('Ctrl Pts',(0.107685092815524,-5.2260494948765,
-1.23492835474597)) ;
#124736=CARTESIAN_POINT('Ctrl Pts',(-0.214157127434278,-5.2042332401232,
-1.22150263084659)) ;
#124737=CARTESIAN_POINT('Ctrl Pts',(-0.374139095164007,-5.19338877303862,
-1.18235894157638)) ;
#124738=CARTESIAN_POINT('Ctrl Pts',(-0.662866899682181,-5.17381719746088,
-1.04700112806878)) ;
#124739=CARTESIAN_POINT('Ctrl Pts',(-0.790050604030013,-5.16468398806342,
-0.954693314448044)) ;
#124740=CARTESIAN_POINT('Ctrl Pts',(-1.00674170146085,-5.14377831804275,
-0.72368004841069)) ;
#124741=CARTESIAN_POINT('Ctrl Pts',(-1.09272499297458,-5.13277145411584,
-0.58582489381677)) ;
#124742=CARTESIAN_POINT('Ctrl Pts',(-1.2024388735119,-5.1120432358759,-0.296071124635525)) ;
#124743=CARTESIAN_POINT('Ctrl Pts',(-1.2293670625,-5.10247198077965,-0.148575526824205)) ;
#124744=CARTESIAN_POINT('Ctrl Pts',(-1.2293670625,-5.09375000068278,8.31973379078477E-14)) ;
#124745=CARTESIAN_POINT('Ctrl Pts',(-1.2293670625,-4.96875000068279,2.28983498828939E-15)) ;
#124746=CARTESIAN_POINT('Ctrl Pts',(-1.2293670625,-4.9779692030022,-0.157045513322919)) ;
#124747=CARTESIAN_POINT('Ctrl Pts',(-1.19927615342303,-4.98813037442379,
-0.312764108202359)) ;
#124748=CARTESIAN_POINT('Ctrl Pts',(-1.08066375780161,-5.00946453554043,
-0.607702317713977)) ;
#124749=CARTESIAN_POINT('Ctrl Pts',(-0.992116119573704,-5.02043967283196,
-0.743536495191188)) ;
#124750=CARTESIAN_POINT('Ctrl Pts',(-0.771076879831951,-5.04123142702765,
-0.970098848476667)) ;
#124751=CARTESIAN_POINT('Ctrl Pts',(-0.642007014364489,-5.05023119644413,
-1.05993767817084)) ;
#124752=CARTESIAN_POINT('Ctrl Pts',(-0.35052171785429,-5.06998969015752,
-1.18957625383883)) ;
#124753=CARTESIAN_POINT('Ctrl Pts',(-0.189775773925879,-5.08088594379565,
-1.22552972972925)) ;
#124754=CARTESIAN_POINT('Ctrl Pts',(0.131982747362557,-5.10269652496808,
-1.23252888345983)) ;
#124755=CARTESIAN_POINT('Ctrl Pts',(0.289899945947995,-5.11340103052236,
-1.20520492820835)) ;
#124756=CARTESIAN_POINT('Ctrl Pts',(0.586151376763805,-5.13348259931309,
-1.09216483808053)) ;
#124757=CARTESIAN_POINT('Ctrl Pts',(0.721719503405525,-5.14238657510161,
-1.00773069578433)) ;
#124758=CARTESIAN_POINT('Ctrl Pts',(0.956960869932357,-5.16321320460779,
-0.788773856918631)) ;
#124759=CARTESIAN_POINT('Ctrl Pts',(1.05302964360807,-5.17432082613859,
-0.65502519170843)) ;
#124760=CARTESIAN_POINT('Ctrl Pts',(1.18484451629919,-5.19590391876801,
-0.363468984722966)) ;
#124761=CARTESIAN_POINT('Ctrl Pts',(1.22153340201252,-5.20619242080942,
-0.209390706018484)) ;
#124762=CARTESIAN_POINT('Ctrl Pts',(1.23524705774866,-5.22547449563549,
0.11115433015815)) ;
#124763=CARTESIAN_POINT('Ctrl Pts',(1.20945802580139,-5.2355482796211,0.274657637770185)) ;
#124764=CARTESIAN_POINT('Ctrl Pts',(1.0962294828551,-5.25726770184908,0.579266988739864)) ;
#124765=CARTESIAN_POINT('Ctrl Pts',(1.0110180947514,-5.2682831804208,0.717714549087699)) ;
#124766=CARTESIAN_POINT('Ctrl Pts',(0.79562688147457,-5.28922234415717,
0.950048855965618)) ;
#124767=CARTESIAN_POINT('Ctrl Pts',(0.668997995129403,-5.29840159772973,
1.04309131886271)) ;
#124768=CARTESIAN_POINT('Ctrl Pts',(0.381093133546937,-5.3179173896607,
1.18013529979385)) ;
#124769=CARTESIAN_POINT('Ctrl Pts',(0.221349534550088,-5.32874569878751,
1.2202190139566)) ;
#124770=CARTESIAN_POINT('Ctrl Pts',(-0.100492620884541,-5.35056194914727,
1.23554610633831)) ;
#124771=CARTESIAN_POINT('Ctrl Pts',(-0.259452092351532,-5.36133710575128,
1.2121755814012)) ;
#124772=CARTESIAN_POINT('Ctrl Pts',(-0.55806114307902,-5.38157848712523,
1.10667077730846)) ;
#124773=CARTESIAN_POINT('Ctrl Pts',(-0.695076546443144,-5.39040120294259,
1.02616841726249)) ;
#124774=CARTESIAN_POINT('Ctrl Pts',(-0.935832077499682,-5.41102695405935,
0.813817067734723)) ;
#124775=CARTESIAN_POINT('Ctrl Pts',(-1.03564439017971,-5.42213148123599,
0.682282446891744)) ;
#124776=CARTESIAN_POINT('Ctrl Pts',(-1.17527171908201,-5.4438177929767,
0.393478466327615)) ;
#124777=CARTESIAN_POINT('Ctrl Pts',(-1.21594161068744,-5.45420657140173,
0.239990453388942)) ;
#124778=CARTESIAN_POINT('Ctrl Pts',(-1.22843447299397,-5.46547080560192,
0.0553213775535472)) ;
#124779=CARTESIAN_POINT('Ctrl Pts',(-1.2293670625,-5.46712701393339,0.0276469458359286)) ;
#124780=CARTESIAN_POINT('Ctrl Pts',(-1.2293670625,-5.46875000068277,3.46253862732339E-13)) ;
#124781=CARTESIAN_POINT('Origin',(0.,-6.,0.)) ;
#124782=CARTESIAN_POINT('',(-5.11233613721112E-18,-5.375,-1.5)) ;
#124783=CARTESIAN_POINT('',(2.44084776499009E-15,-5.43750000136559,-1.5)) ;
#124784=CARTESIAN_POINT('',(-1.83697019872103E-16,-6.,-1.5)) ;
#124785=CARTESIAN_POINT('',(1.5,-5.5,2.18789702550307E-15)) ;
#124786=CARTESIAN_POINT('Ctrl Pts',(2.6028203465122E-16,-5.375,-1.5)) ;
#124787=CARTESIAN_POINT('Ctrl Pts',(0.00627939642630949,-5.37534885535701,
-1.5)) ;
#124788=CARTESIAN_POINT('Ctrl Pts',(0.0125606239867182,-5.37569781244372,
-1.49996056922169)) ;
#124789=CARTESIAN_POINT('Ctrl Pts',(0.211760718905342,-5.38676448438364,
-1.49745797770769)) ;
#124790=CARTESIAN_POINT('Ctrl Pts',(0.402432473209262,-5.39735735962274,
-1.45783659499529)) ;
#124791=CARTESIAN_POINT('Ctrl Pts',(0.759763626140605,-5.41720909034115,
-1.30790067891821)) ;
#124792=CARTESIAN_POINT('Ctrl Pts',(0.922783335544204,-5.42630494071755,
-1.19846684672405)) ;
#124793=CARTESIAN_POINT('Ctrl Pts',(1.20053817819605,-5.44737703217331,
-0.920853483620446)) ;
#124794=CARTESIAN_POINT('Ctrl Pts',(1.31154581317371,-5.45846953542253,
-0.754390421027587)) ;
#124795=CARTESIAN_POINT('Ctrl Pts',(1.46163692622999,-5.48017399618236,
-0.3899268201106)) ;
#124796=CARTESIAN_POINT('Ctrl Pts',(1.49999999999998,-5.4905763386166,-0.195867123712562)) ;
#124797=CARTESIAN_POINT('Ctrl Pts',(1.5,-5.49999999999999,-1.21361254379337E-13)) ;
#124798=CARTESIAN_POINT('',(1.0702882195569,-5.5,-1.05094392194718)) ;
#124799=CARTESIAN_POINT('Origin',(0.,-5.5,0.)) ;
#124800=CARTESIAN_POINT('Ctrl Pts',(1.07028821955797,-5.50000000000008,
-1.05094392194609)) ;
#124801=CARTESIAN_POINT('Ctrl Pts',(0.951434023208664,-5.49087486355005,
-1.17198581917894)) ;
#124802=CARTESIAN_POINT('Ctrl Pts',(0.812952038001049,-5.48266400347676,
-1.27195507031725)) ;
#124803=CARTESIAN_POINT('Ctrl Pts',(0.488455764700654,-5.46463643273785,
-1.43116046170094)) ;
#124804=CARTESIAN_POINT('Ctrl Pts',(0.301613723641133,-5.45425631934565,
-1.48182926271782)) ;
#124805=CARTESIAN_POINT('Ctrl Pts',(0.0735608407828244,-5.44158671474241,
-1.49864874723003)) ;
#124806=CARTESIAN_POINT('Ctrl Pts',(0.0367597598691759,-5.43954221024721,
-1.5)) ;
#124807=CARTESIAN_POINT('Ctrl Pts',(5.8009255759016E-15,-5.43750000136559,
-1.5)) ;
#124808=CARTESIAN_POINT('Origin',(0.,-6.,0.)) ;
#124809=CARTESIAN_POINT('',(-5.60223848449789E-16,-4.875,-1.5)) ;
#124810=CARTESIAN_POINT('',(2.73575075590614E-15,-4.93750000136559,-1.5)) ;
#124811=CARTESIAN_POINT('',(-1.83697019872103E-16,-6.,-1.5)) ;
#124812=CARTESIAN_POINT('Ctrl Pts',(-2.90044460754259E-15,-4.875,-1.5)) ;
#124813=CARTESIAN_POINT('Ctrl Pts',(0.0349268394965454,-4.87694037997203,
-1.5)) ;
#124814=CARTESIAN_POINT('Ctrl Pts',(0.0698921259947087,-4.8788828958886,
-1.4987801389553)) ;
#124815=CARTESIAN_POINT('Ctrl Pts',(0.296235001513499,-4.89145750008409,
-1.48292265504425)) ;
#124816=CARTESIAN_POINT('Ctrl Pts',(0.483325472522242,-4.90185141514013,
-1.43291016146182)) ;
#124817=CARTESIAN_POINT('Ctrl Pts',(0.833833573082252,-4.92132408739346,
-1.26247976005801)) ;
#124818=CARTESIAN_POINT('Ctrl Pts',(0.992890450701865,-4.93098682628875,
-1.14163204431774)) ;
#124819=CARTESIAN_POINT('Ctrl Pts',(1.25436042977266,-4.9524833708566,-0.845794518574959)) ;
#124820=CARTESIAN_POINT('Ctrl Pts',(1.35445596581748,-4.96353065663441,
-0.673971180220349)) ;
#124821=CARTESIAN_POINT('Ctrl Pts',(1.48027440059481,-4.98463133952581,
-0.308043029300386)) ;
#124822=CARTESIAN_POINT('Ctrl Pts',(1.50734151292801,-4.99410432545235,
-0.118300669872091)) ;
#124823=CARTESIAN_POINT('Ctrl Pts',(1.48883164120595,-5.01330273861437,
0.270044174962478)) ;
#124824=CARTESIAN_POINT('Ctrl Pts',(1.43996163357746,-5.02402998059384,
0.464790600505272)) ;
#124825=CARTESIAN_POINT('Ctrl Pts',(1.27095866584812,-5.0458190474935,0.820093942629593)) ;
#124826=CARTESIAN_POINT('Ctrl Pts',(1.15391895956398,-5.05666462066784,
0.977942042002604)) ;
#124827=CARTESIAN_POINT('Ctrl Pts',(0.868676473684781,-5.07708618396317,
1.23771143836587)) ;
#124828=CARTESIAN_POINT('Ctrl Pts',(0.704105023314977,-5.08588305426029,
1.33819376579349)) ;
#124829=CARTESIAN_POINT('Ctrl Pts',(0.337688250459132,-5.10623954164117,
1.47512215716681)) ;
#124830=CARTESIAN_POINT('Ctrl Pts',(0.138187517703181,-5.11732291568316,
1.506953454537)) ;
#124831=CARTESIAN_POINT('Ctrl Pts',(-0.253896032125235,-5.13910533511807,
1.49082395737517)) ;
#124832=CARTESIAN_POINT('Ctrl Pts',(-0.442856428360514,-5.14960313490892,
1.44599994376874)) ;
#124833=CARTESIAN_POINT('Ctrl Pts',(-0.796837488041822,-5.16926874933566,
1.28588072861318)) ;
#124834=CARTESIAN_POINT('Ctrl Pts',(-0.957898920644956,-5.17860925758179,
1.17084651260735)) ;
#124835=CARTESIAN_POINT('Ctrl Pts',(-1.22769099510352,-5.19989497128947,
0.884195788016511)) ;
#124836=CARTESIAN_POINT('Ctrl Pts',(-1.33334132709955,-5.21097013125647,
0.715000158456778)) ;
#124837=CARTESIAN_POINT('Ctrl Pts',(-1.47043879159951,-5.23223468081537,
0.352178053658129)) ;
#124838=CARTESIAN_POINT('Ctrl Pts',(-1.50319554783772,-5.24206769335176,
0.163024947227471)) ;
#124839=CARTESIAN_POINT('Ctrl Pts',(-1.4961573087957,-5.26097674263809,
-0.225928732608051)) ;
#124840=CARTESIAN_POINT('Ctrl Pts',(-1.45307315827811,-5.27160694938967,
-0.421998784973272)) ;
#124841=CARTESIAN_POINT('Ctrl Pts',(-1.2944520114607,-5.29336372026264,
-0.782624813886513)) ;
#124842=CARTESIAN_POINT('Ctrl Pts',(-1.1817196818813,-5.304272525567,-0.944274033501697)) ;
#124843=CARTESIAN_POINT('Ctrl Pts',(-0.904044499744878,-5.32486772741253,
-1.21202142421113)) ;
#124844=CARTESIAN_POINT('Ctrl Pts',(-0.743003475249922,-5.33372202915279,
-1.31690283208648)) ;
#124845=CARTESIAN_POINT('Ctrl Pts',(-0.386661677317576,-5.35351879570459,
-1.46228259539781)) ;
#124846=CARTESIAN_POINT('Ctrl Pts',(-0.194206592983103,-5.36421074483427,
-1.5)) ;
#124847=CARTESIAN_POINT('Ctrl Pts',(3.46944695195361E-16,-5.375,-1.5)) ;
#124848=CARTESIAN_POINT('Ctrl Pts',(5.62050406216485E-15,-5.43750000136559,
-1.5)) ;
#124849=CARTESIAN_POINT('Ctrl Pts',(-0.161994290474594,-5.42850031856145,
-1.5)) ;
#124850=CARTESIAN_POINT('Ctrl Pts',(-0.323186117287328,-5.41954521707184,
-1.47375554236172)) ;
#124851=CARTESIAN_POINT('Ctrl Pts',(-0.659347051983786,-5.4008696095887,
-1.36094099963937)) ;
#124852=CARTESIAN_POINT('Ctrl Pts',(-0.828000153264918,-5.39204971142785,
-1.26543038225483)) ;
#124853=CARTESIAN_POINT('Ctrl Pts',(-1.12165392398143,-5.37182789626481,
-1.01466893042269)) ;
#124854=CARTESIAN_POINT('Ctrl Pts',(-1.24336974114535,-5.36106353363079,
-0.861208514308281)) ;
#124855=CARTESIAN_POINT('Ctrl Pts',(-1.42378561965319,-5.33926125406271,
-0.512219799137908)) ;
#124856=CARTESIAN_POINT('Ctrl Pts',(-1.47908425176341,-5.32843676932294,
-0.319163788852183)) ;
#124857=CARTESIAN_POINT('Ctrl Pts',(-1.51042735663741,-5.30892123156154,
0.0683630963888204)) ;
#124858=CARTESIAN_POINT('Ctrl Pts',(-1.48965804817001,-5.2997591131944,
0.258843459079508)) ;
#124859=CARTESIAN_POINT('Ctrl Pts',(-1.37625164813583,-5.2788448851852,
0.628062309648105)) ;
#124860=CARTESIAN_POINT('Ctrl Pts',(-1.28234235921275,-5.26784005660849,
0.802574823090399)) ;
#124861=CARTESIAN_POINT('Ctrl Pts',(-1.0302400818302,-5.24612128021888,
1.10843979560054)) ;
#124862=CARTESIAN_POINT('Ctrl Pts',(-0.873405472831508,-5.23602252763399,
1.23578325781099)) ;
#124863=CARTESIAN_POINT('Ctrl Pts',(-0.526771579872414,-5.21676508913627,
1.41743721034463)) ;
#124864=CARTESIAN_POINT('Ctrl Pts',(-0.341867333422598,-5.20649263100017,
1.47299730884172)) ;
#124865=CARTESIAN_POINT('Ctrl Pts',(0.0462100909223037,-5.18493277409212,
1.51240764724932)) ;
#124866=CARTESIAN_POINT('Ctrl Pts',(0.246014476734837,-5.17383253043587,
1.49298285093653)) ;
#124867=CARTESIAN_POINT('Ctrl Pts',(0.621002890592565,-5.15299984077711,
1.37900479354308)) ;
#124868=CARTESIAN_POINT('Ctrl Pts',(0.793171709133358,-5.14408867506976,
1.28770123413088)) ;
#124869=CARTESIAN_POINT('Ctrl Pts',(1.09381042503216,-5.12403797775275,
1.04452915992086)) ;
#124870=CARTESIAN_POINT('Ctrl Pts',(1.21930985636277,-5.11334977285415,
0.894836123269743)) ;
#124871=CARTESIAN_POINT('Ctrl Pts',(1.40907773114056,-5.0915550033271,0.551402878935084)) ;
#124872=CARTESIAN_POINT('Ctrl Pts',(1.46969977226217,-5.08065861913372,
0.359925938194671)) ;
#124873=CARTESIAN_POINT('Ctrl Pts',(1.51176058718588,-5.06088381495732,
-0.0268018255058508)) ;
#124874=CARTESIAN_POINT('Ctrl Pts',(1.49620870472285,-5.05190795725008,
-0.217962597419856)) ;
#124875=CARTESIAN_POINT('Ctrl Pts',(1.39300652386959,-5.03115159167009,
-0.589791747703553)) ;
#124876=CARTESIAN_POINT('Ctrl Pts',(1.30423149612885,-5.02019081729288,
-0.76635287887949)) ;
#124877=CARTESIAN_POINT('Ctrl Pts',(1.06197871256978,-4.9984749914188,-1.07784313398654)) ;
#124878=CARTESIAN_POINT('Ctrl Pts',(0.909936830813567,-4.98805204752189,
-1.20892691786967)) ;
#124879=CARTESIAN_POINT('Ctrl Pts',(0.57067768749066,-4.96920431733728,
-1.40025758894091)) ;
#124880=CARTESIAN_POINT('Ctrl Pts',(0.388176202716192,-4.95906534596093,
-1.46139985085397)) ;
#124881=CARTESIAN_POINT('Ctrl Pts',(0.132995506608445,-4.94488864062161,
-1.49558275095357)) ;
#124882=CARTESIAN_POINT('Ctrl Pts',(0.0664632989529273,-4.94119240686297,
-1.5)) ;
#124883=CARTESIAN_POINT('Ctrl Pts',(6.54463398306847E-15,-4.93750000136559,
-1.5)) ;
#124884=CARTESIAN_POINT('Origin',(0.,-6.,0.)) ;
#124885=CARTESIAN_POINT('',(-2.58117669796277E-15,-4.375,-1.5)) ;
#124886=CARTESIAN_POINT('',(-1.94691842705875E-15,-4.43750000136559,-1.5)) ;
#124887=CARTESIAN_POINT('',(-1.83697019872103E-16,-6.,-1.5)) ;
#124888=CARTESIAN_POINT('Ctrl Pts',(-2.90044460754259E-15,-4.375,-1.5)) ;
#124889=CARTESIAN_POINT('Ctrl Pts',(0.0646412971543186,-4.37859118317524,
-1.5)) ;
#124890=CARTESIAN_POINT('Ctrl Pts',(0.129351575045616,-4.38218619861364,
-1.49582161897791)) ;
#124891=CARTESIAN_POINT('Ctrl Pts',(0.382903534036573,-4.39627241855758,
-1.46279893074578)) ;
#124892=CARTESIAN_POINT('Ctrl Pts',(0.565688061329142,-4.40642711451828,
-1.40228980244635)) ;
#124893=CARTESIAN_POINT('Ctrl Pts',(0.9056869803183,-4.42531594335101,-1.21211601328188)) ;
#124894=CARTESIAN_POINT('Ctrl Pts',(1.0581933129685,-4.43569097384046,-1.08156079863571)) ;
#124895=CARTESIAN_POINT('Ctrl Pts',(1.30158022961293,-4.45740012168722,
-0.770864135762298)) ;
#124896=CARTESIAN_POINT('Ctrl Pts',(1.39099228872664,-4.46836678784929,
-0.594548336372274)) ;
#124897=CARTESIAN_POINT('Ctrl Pts',(1.49545643839563,-4.4891428936166,-0.223037492035378)) ;
#124898=CARTESIAN_POINT('Ctrl Pts',(1.51165586675903,-4.49813833108958,
-0.0319645438657472)) ;
#124899=CARTESIAN_POINT('Ctrl Pts',(1.47092876716576,-4.51788115719622,
0.354868589041279)) ;
#124900=CARTESIAN_POINT('Ctrl Pts',(1.41096661834321,-4.52876906002735,
0.546550236973955)) ;
#124901=CARTESIAN_POINT('Ctrl Pts',(1.22235311022667,-4.55056568182347,
0.890688453901026)) ;
#124902=CARTESIAN_POINT('Ctrl Pts',(1.09731829876053,-4.56126377194236,
1.04085519940139)) ;
#124903=CARTESIAN_POINT('Ctrl Pts',(0.797546755734701,-4.58133598597994,
1.28497515274195)) ;
#124904=CARTESIAN_POINT('Ctrl Pts',(0.625821141799246,-4.59023215878893,
1.37680518623772)) ;
#124905=CARTESIAN_POINT('Ctrl Pts',(0.251311008607692,-4.61103827729958,
1.4921099010432)) ;
#124906=CARTESIAN_POINT('Ctrl Pts',(0.0515039259646006,-4.62213867077975,
1.5122458642563)) ;
#124907=CARTESIAN_POINT('Ctrl Pts',(-0.336840442440354,-4.64371335791335,
1.47416320532842)) ;
#124908=CARTESIAN_POINT('Ctrl Pts',(-0.521994293529454,-4.65399968297386,
1.41921195969608)) ;
#124909=CARTESIAN_POINT('Ctrl Pts',(-0.86906205182113,-4.67328122510117,
1.23880073999231)) ;
#124910=CARTESIAN_POINT('Ctrl Pts',(-1.0261453300444,-4.68332733239396,
1.11218525198224)) ;
#124911=CARTESIAN_POINT('Ctrl Pts',(-1.27930114605304,-4.70502190906147,
0.807431522059718)) ;
#124912=CARTESIAN_POINT('Ctrl Pts',(-1.37390227146845,-4.71603206906703,
0.633207628934896)) ;
#124913=CARTESIAN_POINT('Ctrl Pts',(-1.48868992421953,-4.7369673532902,
0.264348599805235)) ;
#124914=CARTESIAN_POINT('Ctrl Pts',(-1.51016244923422,-4.74615954009191,
0.0739551674221457)) ;
#124915=CARTESIAN_POINT('Ctrl Pts',(-1.4802584543877,-4.76563987235946,
-0.313670855932048)) ;
#124916=CARTESIAN_POINT('Ctrl Pts',(-1.42567798733999,-4.77645405423592,
-0.506927358017484)) ;
#124917=CARTESIAN_POINT('Ctrl Pts',(-1.24653064568719,-4.79825605774633,
-0.856642725531518)) ;
#124918=CARTESIAN_POINT('Ctrl Pts',(-1.12533143605636,-4.80903007223487,
-1.01060201517332)) ;
#124919=CARTESIAN_POINT('Ctrl Pts',(-0.832618460366114,-4.82927455266081,
-1.26237772390985)) ;
#124920=CARTESIAN_POINT('Ctrl Pts',(-0.664429502277172,-4.8380872498735,
-1.3584494122206)) ;
#124921=CARTESIAN_POINT('Ctrl Pts',(-0.327003075299122,-4.85683316248339,
-1.47312623171267)) ;
#124922=CARTESIAN_POINT('Ctrl Pts',(-0.163924989693454,-4.86589305612814,
-1.5)) ;
#124923=CARTESIAN_POINT('Ctrl Pts',(-3.46944695195361E-15,-4.875,-1.5)) ;
#124924=CARTESIAN_POINT('Ctrl Pts',(6.69603261727048E-15,-4.93750000136559,
-1.5)) ;
#124925=CARTESIAN_POINT('Ctrl Pts',(-0.130815870223861,-4.93023245301982,
-1.5)) ;
#124926=CARTESIAN_POINT('Ctrl Pts',(-0.261364789692205,-4.92297973527157,
-1.48288628464552)) ;
#124927=CARTESIAN_POINT('Ctrl Pts',(-0.576211118206899,-4.90548827257631,
-1.39851230341137)) ;
#124928=CARTESIAN_POINT('Ctrl Pts',(-0.752521316565833,-4.89639089959295,
-1.31208255717432)) ;
#124929=CARTESIAN_POINT('Ctrl Pts',(-1.06108752372491,-4.87654051230214,
-1.07765078788927)) ;
#124930=CARTESIAN_POINT('Ctrl Pts',(-1.19076365958232,-4.86594830373867,
-0.932364419078407)) ;
#124931=CARTESIAN_POINT('Ctrl Pts',(-1.39186582163854,-4.84408722415966,
-0.594096800006323)) ;
#124932=CARTESIAN_POINT('Ctrl Pts',(-1.45876423175756,-4.83302620311843,
-0.402821609972903)) ;
#124933=CARTESIAN_POINT('Ctrl Pts',(-1.51197026583597,-4.81290441323619,
-0.0153165790875582)) ;
#124934=CARTESIAN_POINT('Ctrl Pts',(-1.50170161487065,-4.80405079988388,
0.176595782800065)) ;
#124935=CARTESIAN_POINT('Ctrl Pts',(-1.40874187252435,-4.78345686103223,
0.550962431560849)) ;
#124936=CARTESIAN_POINT('Ctrl Pts',(-1.32515569478117,-4.77254848933251,
0.729430177481386)) ;
#124937=CARTESIAN_POINT('Ctrl Pts',(-1.09222653520524,-4.75079140970906,
1.04716087248384)) ;
#124938=CARTESIAN_POINT('Ctrl Pts',(-0.943996237490369,-4.74016045303707,
1.18254035526347)) ;
#124939=CARTESIAN_POINT('Ctrl Pts',(-0.610717416559541,-4.72124925036386,
1.38318370463077)) ;
#124940=CARTESIAN_POINT('Ctrl Pts',(-0.430545184352667,-4.71141917827407,
1.44943066767392)) ;
#124941=CARTESIAN_POINT('Ctrl Pts',(-0.0478048447914621,-4.69015582607623,
1.51219616926508)) ;
#124942=CARTESIAN_POINT('Ctrl Pts',(0.151544985468626,-4.67908083550622,
1.50534371639794)) ;
#124943=CARTESIAN_POINT('Ctrl Pts',(0.534716566927561,-4.65779352542517,
1.41510953087164)) ;
#124944=CARTESIAN_POINT('Ctrl Pts',(0.714899541237845,-4.64845088828263,
1.3331776759439)) ;
#124945=CARTESIAN_POINT('Ctrl Pts',(1.03061126520019,-4.62878669835578,
1.10674141224403)) ;
#124946=CARTESIAN_POINT('Ctrl Pts',(1.16393729767628,-4.61828964652437,
0.965540107763861)) ;
#124947=CARTESIAN_POINT('Ctrl Pts',(1.37401459251156,-4.59650789075635,
0.634102998468438)) ;
#124948=CARTESIAN_POINT('Ctrl Pts',(1.4462381198111,-4.58542438206486,0.445434869239173)) ;
#124949=CARTESIAN_POINT('Ctrl Pts',(1.5109498623578,-4.56506613345469,0.0596579598670437)) ;
#124950=CARTESIAN_POINT('Ctrl Pts',(1.50625743322842,-4.55626941762015,
-0.133112982053908)) ;
#124951=CARTESIAN_POINT('Ctrl Pts',(1.42399202102172,-4.5358491728675,-0.510043841146295)) ;
#124952=CARTESIAN_POINT('Ctrl Pts',(1.34585236191532,-4.52500410689068,
-0.690340351326157)) ;
#124953=CARTESIAN_POINT('Ctrl Pts',(1.12272623748609,-4.5032148709766,-1.01439918725928)) ;
#124954=CARTESIAN_POINT('Ctrl Pts',(0.978536665193565,-4.49248693785947,
-1.15412720151065)) ;
#124955=CARTESIAN_POINT('Ctrl Pts',(0.651522387758622,-4.47328637770086,
-1.36440156914687)) ;
#124956=CARTESIAN_POINT('Ctrl Pts',(0.473684284235579,-4.46381579493424,
-1.43587098432322)) ;
#124957=CARTESIAN_POINT('Ctrl Pts',(0.192349898494841,-4.44818610683753,
-1.49075118620303)) ;
#124958=CARTESIAN_POINT('Ctrl Pts',(0.0961708540385476,-4.44284282658996,
-1.5)) ;
#124959=CARTESIAN_POINT('Ctrl Pts',(-3.27231699153423E-15,-4.43750000136559,
-1.5)) ;
#124960=CARTESIAN_POINT('Origin',(0.,-6.,0.)) ;
#124961=CARTESIAN_POINT('',(1.4076030946114E-15,-3.875,-1.5)) ;
#124962=CARTESIAN_POINT('',(-1.51432176023703E-15,-3.93750000136559,-1.5)) ;
#124963=CARTESIAN_POINT('',(-1.83697019872103E-16,-6.,-1.5)) ;
#124964=CARTESIAN_POINT('Ctrl Pts',(2.60282034651221E-16,-3.875,-1.5)) ;
#124965=CARTESIAN_POINT('Ctrl Pts',(0.0942423192034461,-3.88023568440019,
-1.5)) ;
#124966=CARTESIAN_POINT('Ctrl Pts',(0.188500951634548,-3.8854722750908,
-1.4911184271582)) ;
#124967=CARTESIAN_POINT('Ctrl Pts',(0.46816646802523,-3.90100924822362,
-1.43768292334024)) ;
#124968=CARTESIAN_POINT('Ctrl Pts',(0.646300575696504,-3.91052180730236,
-1.36688571863216)) ;
#124969=CARTESIAN_POINT('Ctrl Pts',(0.974128090628617,-3.92968536543257,
-1.15784994660216)) ;
#124970=CARTESIAN_POINT('Ctrl Pts',(1.11884638083205,-3.94040132656015,
-1.01867602090901)) ;
#124971=CARTESIAN_POINT('Ctrl Pts',(1.34324687246104,-3.96218750156777,
-0.695416560967739)) ;
#124972=CARTESIAN_POINT('Ctrl Pts',(1.42209117090439,-3.97304122919988,
-0.5153468453742)) ;
#124973=CARTESIAN_POINT('Ctrl Pts',(1.50573756977115,-3.99348413465912,
-0.138742305359965)) ;
#124974=CARTESIAN_POINT('Ctrl Pts',(1.51115389055952,-4.00228408629164,
0.0539135437891495)) ;
#124975=CARTESIAN_POINT('Ctrl Pts',(1.44793534887079,-4.02261199480333,
0.439921945973768)) ;
#124976=CARTESIAN_POINT('Ctrl Pts',(1.3763982541349,-4.03369311341226,0.628936710295236)) ;
#124977=CARTESIAN_POINT('Ctrl Pts',(1.16747431042337,-4.05548614561118,
0.961274083387404)) ;
#124978=CARTESIAN_POINT('Ctrl Pts',(1.03461530485744,-4.0659959981852,1.10301108441868)) ;
#124979=CARTESIAN_POINT('Ctrl Pts',(0.719830412477448,-4.08568464584996,
1.33049079911853)) ;
#124980=CARTESIAN_POINT('Ctrl Pts',(0.540157294751756,-4.09499126140268,
1.41301220964346)) ;
#124981=CARTESIAN_POINT('Ctrl Pts',(0.157480541459988,-4.11625108103,1.50474454179345)) ;
#124982=CARTESIAN_POINT('Ctrl Pts',(-0.041920265696383,-4.1273289036498,
1.51238076232928)) ;
#124983=CARTESIAN_POINT('Ctrl Pts',(-0.425030160643521,-4.14861278670241,
1.4510648450455)) ;
#124984=CARTESIAN_POINT('Ctrl Pts',(-0.605504207978813,-4.15849392757573,
1.3854806133664)) ;
#124985=CARTESIAN_POINT('Ctrl Pts',(-0.939569016813357,-4.17736812341821,
1.18606022685966)) ;
#124986=CARTESIAN_POINT('Ctrl Pts',(-1.08830077291439,-4.18798613601125,
1.05123929884302)) ;
#124987=CARTESIAN_POINT('Ctrl Pts',(-1.3224570684676,-4.20973777009996,
0.734330274441642)) ;
#124988=CARTESIAN_POINT('Ctrl Pts',(-1.40672934906018,-4.2206535178302,
0.556105342270486)) ;
#124989=CARTESIAN_POINT('Ctrl Pts',(-1.50103999144478,-4.2412691022799,
0.182068740703184)) ;
#124990=CARTESIAN_POINT('Ctrl Pts',(-1.51200845611127,-4.25013507314821,
-0.00974052803380514)) ;
#124991=CARTESIAN_POINT('Ctrl Pts',(-1.46024638357755,-4.27022676020464,
-0.397453555020732)) ;
#124992=CARTESIAN_POINT('Ctrl Pts',(-1.39402190482696,-4.28128429938543,
-0.589045470400813)) ;
#124993=CARTESIAN_POINT('Ctrl Pts',(-1.19406008533681,-4.30315410409528,
-0.928152814999461)) ;
#124994=CARTESIAN_POINT('Ctrl Pts',(-1.06485019338996,-4.31375768718844,
-1.07394478501753)) ;
#124995=CARTESIAN_POINT('Ctrl Pts',(-0.757181391102665,-4.3336310782375,
-1.3093727953836)) ;
#124996=CARTESIAN_POINT('Ctrl Pts',(-0.581348167225834,-4.34270287959856,
-1.39636008114215)) ;
#124997=CARTESIAN_POINT('Ctrl Pts',(-0.265154173659441,-4.36026921257447,
-1.48238373539969)) ;
#124998=CARTESIAN_POINT('Ctrl Pts',(-0.132722487609192,-4.36762652846615,
-1.5)) ;
#124999=CARTESIAN_POINT('Ctrl Pts',(-3.01841884819964E-15,-4.375,-1.5)) ;
#125000=CARTESIAN_POINT('Ctrl Pts',(-3.97251675998689E-15,-4.43750000136559,
-1.5)) ;
#125001=CARTESIAN_POINT('Ctrl Pts',(-0.0998335372168724,-4.43195369374243,
-1.5)) ;
#125002=CARTESIAN_POINT('Ctrl Pts',(-0.199658248269081,-4.42640787646175,
-1.49003323466658)) ;
#125003=CARTESIAN_POINT('Ctrl Pts',(-0.49191789941691,-4.41017122917576,
-1.43079611298183)) ;
#125004=CARTESIAN_POINT('Ctrl Pts',(-0.676133757207218,-4.40050582845571,
-1.35350736953389)) ;
#125005=CARTESIAN_POINT('Ctrl Pts',(-0.999037892355418,-4.38103459961541,
-1.13523426723781)) ;
#125006=CARTESIAN_POINT('Ctrl Pts',(-1.1359209996514,-4.37064148043957,
-0.998246840542587)) ;
#125007=CARTESIAN_POINT('Ctrl Pts',(-1.35483349461492,-4.34895721561397,
-0.673937047606172)) ;
#125008=CARTESIAN_POINT('Ctrl Pts',(-1.43233728352691,-4.33786052119468,
-0.488043418634293)) ;
#125009=CARTESIAN_POINT('Ctrl Pts',(-1.50864480205144,-4.31727026199915,
-0.104139084183682)) ;
#125010=CARTESIAN_POINT('Ctrl Pts',(-1.50958033404375,-4.30845717980767,
0.0895596765701229)) ;
#125011=CARTESIAN_POINT('Ctrl Pts',(-1.43797083262724,-4.28821401126395,
0.468962268737551)) ;
#125012=CARTESIAN_POINT('Ctrl Pts',(-1.36527778751035,-4.27744055255317,
0.650915053894818)) ;
#125013=CARTESIAN_POINT('Ctrl Pts',(-1.15206224529449,-4.25563852472727,
0.980961642031033)) ;
#125014=CARTESIAN_POINT('Ctrl Pts',(-1.0120182649773,-4.24482374142398,
1.12488826214615)) ;
#125015=CARTESIAN_POINT('Ctrl Pts',(-0.691322923457565,-4.22534136580834,
1.34466829341293)) ;
#125016=CARTESIAN_POINT('Ctrl Pts',(-0.515717164638227,-4.2161509549566,
1.42130708291937)) ;
#125017=CARTESIAN_POINT('Ctrl Pts',(-0.138904002513243,-4.1952168903941,
1.5064074405763)) ;
#125018=CARTESIAN_POINT('Ctrl Pts',(0.0592733838908032,-4.18420703559388,
1.511635564)) ;
#125019=CARTESIAN_POINT('Ctrl Pts',(0.449801105031135,-4.16251105108608,
1.44485818892842)) ;
#125020=CARTESIAN_POINT('Ctrl Pts',(0.638024314217126,-4.1524619170851,
1.37216141104746)) ;
#125021=CARTESIAN_POINT('Ctrl Pts',(0.967848797712361,-4.13318177246089,
1.16185538458189)) ;
#125022=CARTESIAN_POINT('Ctrl Pts',(1.10803832240908,-4.12289624965393,
1.02901326739432)) ;
#125023=CARTESIAN_POINT('Ctrl Pts',(1.3352501696126,-4.10132241697745,0.711790396824513)) ;
#125024=CARTESIAN_POINT('Ctrl Pts',(1.41775118270551,-4.09022202847339,
0.528705136468632)) ;
#125025=CARTESIAN_POINT('Ctrl Pts',(1.50523004438318,-4.06941436417902,
0.146731899870329)) ;
#125026=CARTESIAN_POINT('Ctrl Pts',(1.51160504407379,-4.06051734841374,
-0.0479088430764911)) ;
#125027=CARTESIAN_POINT('Ctrl Pts',(1.4501496273714,-4.04044638316897,-0.429594720430866)) ;
#125028=CARTESIAN_POINT('Ctrl Pts',(1.38265615327964,-4.02974886441085,
-0.612971097043189)) ;
#125029=CARTESIAN_POINT('Ctrl Pts',(1.17899944361955,-4.00795234313619,
-0.948422028210402)) ;
#125030=CARTESIAN_POINT('Ctrl Pts',(1.04300877637827,-3.99706394374256,
-1.09621891142586)) ;
#125031=CARTESIAN_POINT('Ctrl Pts',(0.728409026090832,-3.97731925686015,
-1.3249702712289)) ;
#125032=CARTESIAN_POINT('Ctrl Pts',(0.554849708907109,-3.96832498519377,
-1.40651277173017)) ;
#125033=CARTESIAN_POINT('Ctrl Pts',(0.249253928268807,-3.95134744182497,
-1.4844418180471)) ;
#125034=CARTESIAN_POINT('Ctrl Pts',(0.124729698084853,-3.94442942903697,
-1.5)) ;
#125035=CARTESIAN_POINT('Ctrl Pts',(-3.40005801291454E-15,-3.93750000136559,
-1.5)) ;
#125036=CARTESIAN_POINT('Origin',(0.,-6.,0.)) ;
#125037=CARTESIAN_POINT('',(3.08703225979145E-15,-3.37499999999999,-1.5)) ;
#125038=CARTESIAN_POINT('',(-1.32350217787958E-15,-3.43750000136559,-1.5)) ;
#125039=CARTESIAN_POINT('',(-1.83697019872103E-16,-6.,-1.5)) ;
#125040=CARTESIAN_POINT('Ctrl Pts',(1.20736753927986E-14,-3.37499999999999,
-1.5)) ;
#125041=CARTESIAN_POINT('Ctrl Pts',(0.123025767620368,-3.38183476486779,
-1.5)) ;
#125042=CARTESIAN_POINT('Ctrl Pts',(0.245864401420877,-3.38865913341226,
-1.48486403806509)) ;
#125043=CARTESIAN_POINT('Ctrl Pts',(0.550039486660369,-3.4055577492589,
-1.40839677588521)) ;
#125044=CARTESIAN_POINT('Ctrl Pts',(0.723848898809359,-3.41457268167444,
-1.32746242112634)) ;
#125045=CARTESIAN_POINT('Ctrl Pts',(1.03920974331056,-3.43428512761029,
-1.0998205947628)) ;
#125046=CARTESIAN_POINT('Ctrl Pts',(1.17570902074221,-3.44516487040949,
-0.952497281714251)) ;
#125047=CARTESIAN_POINT('Ctrl Pts',(1.38055843843326,-3.46696300706962,
-0.61770138569343)) ;
#125048=CARTESIAN_POINT('Ctrl Pts',(1.44869790488294,-3.47767035854733,
-0.434493603703968)) ;
#125049=CARTESIAN_POINT('Ctrl Pts',(1.5114145116643,-3.49776290479369,-0.053087322086436)) ;
#125050=CARTESIAN_POINT('Ctrl Pts',(1.50571947322053,-3.50664582679239,
0.141433055356179)) ;
#125051=CARTESIAN_POINT('Ctrl Pts',(1.41963444045046,-3.5274267144909,0.523654478355581)) ;
#125052=CARTESIAN_POINT('Ctrl Pts',(1.33775190161653,-3.53852712433378,
0.707097258510357)) ;
#125053=CARTESIAN_POINT('Ctrl Pts',(1.11156381318303,-3.56011561436665,
1.02521584391335)) ;
#125054=CARTESIAN_POINT('Ctrl Pts',(0.971780230466467,-3.57041495677473,
1.15857956682781)) ;
#125055=CARTESIAN_POINT('Ctrl Pts',(0.642818743148598,-3.58971922767343,
1.3698852995673)) ;
#125056=CARTESIAN_POINT('Ctrl Pts',(0.455102019190075,-3.59971655448944,
1.44316189862217)) ;
#125057=CARTESIAN_POINT('Ctrl Pts',(0.0650132634678198,-3.62138815202956,
1.51140914512229)) ;
#125058=CARTESIAN_POINT('Ctrl Pts',(-0.133257745415366,-3.63240320807863,
1.50692689389207)) ;
#125059=CARTESIAN_POINT('Ctrl Pts',(-0.510449552502788,-3.65335830847237,
1.42320674145113)) ;
#125060=CARTESIAN_POINT('Ctrl Pts',(-0.686332998975074,-3.66257994297825,
1.34722090227418)) ;
#125061=CARTESIAN_POINT('Ctrl Pts',(-1.0078327000363,-3.68202700523824,
1.12863924251933)) ;
#125062=CARTESIAN_POINT('Ctrl Pts',(-1.14840782613823,-3.69283133527332,
0.985236546665589)) ;
#125063=CARTESIAN_POINT('Ctrl Pts',(-1.36288531483847,-3.71463279978794,
0.655930251877055)) ;
#125064=CARTESIAN_POINT('Ctrl Pts',(-1.43626868098597,-3.72541578717667,
0.474177973900462)) ;
#125065=CARTESIAN_POINT('Ctrl Pts',(-1.50922719478472,-3.74568156538545,
0.0950843013314755)) ;
#125066=CARTESIAN_POINT('Ctrl Pts',(-1.50900853204741,-3.75448856214089,
-0.0984940905742062)) ;
#125067=CARTESIAN_POINT('Ctrl Pts',(-1.4341764099549,-3.77504963836379,
-0.482643688856358)) ;
#125068=CARTESIAN_POINT('Ctrl Pts',(-1.3573393155221,-3.78614518417671,
-0.66889836072996)) ;
#125069=CARTESIAN_POINT('Ctrl Pts',(-1.13953871385644,-3.80784282577407,
-0.994128136541216)) ;
#125070=CARTESIAN_POINT('Ctrl Pts',(-1.00310120634842,-3.81824961031078,
-1.13165685958585)) ;
#125071=CARTESIAN_POINT('Ctrl Pts',(-0.681111648821587,-3.83774569029164,
-1.35097451477486)) ;
#125072=CARTESIAN_POINT('Ctrl Pts',(-0.497416098316471,-3.84736577231575,
-1.42886065532683)) ;
#125073=CARTESIAN_POINT('Ctrl Pts',(-0.203658757535048,-3.86368562458138,
-1.48962877654428)) ;
#125074=CARTESIAN_POINT('Ctrl Pts',(-0.101838903337983,-3.86934228314789,
-1.5)) ;
#125075=CARTESIAN_POINT('Ctrl Pts',(-6.93889390390723E-17,-3.875,-1.5)) ;
#125076=CARTESIAN_POINT('Ctrl Pts',(-3.27231699153424E-15,-3.93750000136559,
-1.5)) ;
#125077=CARTESIAN_POINT('Ctrl Pts',(-0.070231194483588,-3.93359826833872,
-1.5)) ;
#125078=CARTESIAN_POINT('Ctrl Pts',(-0.140527531456689,-3.92969291628466,
-1.49506770113817)) ;
#125079=CARTESIAN_POINT('Ctrl Pts',(-0.407265219101565,-3.91487415585995,
-1.45728574992466)) ;
#125080=CARTESIAN_POINT('Ctrl Pts',(-0.596595698355777,-3.9044963629537,
-1.3905277518438)) ;
#125081=CARTESIAN_POINT('Ctrl Pts',(-0.931327375415623,-3.88560991898453,
-1.19123780935363)) ;
#125082=CARTESIAN_POINT('Ctrl Pts',(-1.07514580432589,-3.87545613444443,
-1.06322896944864)) ;
#125083=CARTESIAN_POINT('Ctrl Pts',(-1.31157428121161,-3.85402811525593,
-0.754357998942086)) ;
#125084=CARTESIAN_POINT('Ctrl Pts',(-1.39967070126838,-3.8429343023808,
-0.574639920183848)) ;
#125085=CARTESIAN_POINT('Ctrl Pts',(-1.4999169296833,-3.82188614237405,
-0.195039316694249)) ;
#125086=CARTESIAN_POINT('Ctrl Pts',(-1.5125422847797,-3.81281288352773,
0.000738157874615904)) ;
#125087=CARTESIAN_POINT('Ctrl Pts',(-1.46256638272007,-3.79294082983558,
0.384917437113829)) ;
#125088=CARTESIAN_POINT('Ctrl Pts',(-1.40095083835048,-3.78233790561831,
0.569721327423226)) ;
#125089=CARTESIAN_POINT('Ctrl Pts',(-1.2073316710414,-3.76046860146178,
0.912480200160393)) ;
#125090=CARTESIAN_POINT('Ctrl Pts',(-1.07455600022974,-3.749410855499,1.06565306477226)) ;
#125091=CARTESIAN_POINT('Ctrl Pts',(-0.764720191675931,-3.72931741291523,
1.30440363874785)) ;
#125092=CARTESIAN_POINT('Ctrl Pts',(-0.593139462781269,-3.72045219374233,
1.39084758505053)) ;
#125093=CARTESIAN_POINT('Ctrl Pts',(-0.222081613845145,-3.69983786880143,
1.49626828321634)) ;
#125094=CARTESIAN_POINT('Ctrl Pts',(-0.0256058221544604,-3.68892254704084,
1.51244053751281)) ;
#125095=CARTESIAN_POINT('Ctrl Pts',(0.365929456853119,-3.66717058709597,
1.46819562366311)) ;
#125096=CARTESIAN_POINT('Ctrl Pts',(0.557067337200572,-3.65655181596556,
1.40684216814683)) ;
#125097=CARTESIAN_POINT('Ctrl Pts',(0.896841729089794,-3.6376754608606,
1.21731903993412)) ;
#125098=CARTESIAN_POINT('Ctrl Pts',(1.04390101088138,-3.62779733095075,
1.09385063513606)) ;
#125099=CARTESIAN_POINT('Ctrl Pts',(1.28861960359674,-3.60651464312407,
0.792786620866651)) ;
#125100=CARTESIAN_POINT('Ctrl Pts',(1.38174500714516,-3.5954369811341,0.61630771692526)) ;
#125101=CARTESIAN_POINT('Ctrl Pts',(1.4937309636147,-3.5741755542344,0.239052379458141)) ;
#125102=CARTESIAN_POINT('Ctrl Pts',(1.51214651100827,-3.56486686984892,
0.0421816462151671)) ;
#125103=CARTESIAN_POINT('Ctrl Pts',(1.47261553235169,-3.545179647906,-0.344186356596442)) ;
#125104=CARTESIAN_POINT('Ctrl Pts',(1.41633790577741,-3.53467053911417,
-0.530122178180987)) ;
#125105=CARTESIAN_POINT('Ctrl Pts',(1.23306641992855,-3.51287815733459,
-0.877256486013357)) ;
#125106=CARTESIAN_POINT('Ctrl Pts',(1.10518091116016,-3.50179689482562,
-1.03374146923098)) ;
#125107=CARTESIAN_POINT('Ctrl Pts',(0.802552349766301,-3.48146721179632,
-1.28156331474823)) ;
#125108=CARTESIAN_POINT('Ctrl Pts',(0.633014668514489,-3.47266748294973,
-1.37324051716546)) ;
#125109=CARTESIAN_POINT('Ctrl Pts',(0.304714521415647,-3.45442858588868,
-1.47668899033705)) ;
#125110=CARTESIAN_POINT('Ctrl Pts',(0.152673453390108,-3.44598185988726,
-1.5)) ;
#125111=CARTESIAN_POINT('Ctrl Pts',(4.5102810375397E-16,-3.43750000136559,
-1.5)) ;
#125112=CARTESIAN_POINT('Origin',(0.,-6.,0.)) ;
#125113=CARTESIAN_POINT('',(-3.50058014023048E-15,-2.875,-1.5)) ;
#125114=CARTESIAN_POINT('',(-7.16348961287702E-16,-2.93750000136559,-1.5)) ;
#125115=CARTESIAN_POINT('',(-1.83697019872103E-16,-6.,-1.5)) ;
#125116=CARTESIAN_POINT('Ctrl Pts',(-1.3912482277334E-14,-2.875,-1.5)) ;
#125117=CARTESIAN_POINT('Ctrl Pts',(0.14927646169187,-2.88329313676066,
-1.5)) ;
#125118=CARTESIAN_POINT('Ctrl Pts',(0.298008422113359,-2.89155602345074,
-1.47771475584672)) ;
#125119=CARTESIAN_POINT('Ctrl Pts',(0.625668423501798,-2.90975935686121,
-1.37687521093521)) ;
#125120=CARTESIAN_POINT('Ctrl Pts',(0.797408078633453,-2.91865598955823,
-1.28506187278717)) ;
#125121=CARTESIAN_POINT('Ctrl Pts',(1.09720715239368,-2.93872752168036,
-1.04097198767013)) ;
#125122=CARTESIAN_POINT('Ctrl Pts',(1.2222567372371,-2.94942529983834,-0.890820255568953)) ;
#125123=CARTESIAN_POINT('Ctrl Pts',(1.41090692411199,-2.97122186685069,
-0.546704353792156)) ;
#125124=CARTESIAN_POINT('Ctrl Pts',(1.47089002802769,-2.98211004090072,
-0.35502916710887)) ;
#125125=CARTESIAN_POINT('Ctrl Pts',(1.51165945654184,-3.00185388317589,
0.0318006478503855)) ;
#125126=CARTESIAN_POINT('Ctrl Pts',(1.49548058650827,-3.01084868359775,
0.222876369642636)) ;
#125127=CARTESIAN_POINT('Ctrl Pts',(1.39105652263104,-3.03162416325971,
0.594397344166714)) ;
#125128=CARTESIAN_POINT('Ctrl Pts',(1.3016646900582,-3.04259064418931,0.770720971371029)) ;
#125129=CARTESIAN_POINT('Ctrl Pts',(1.0583137636934,-3.06430000807502,1.08144290352728)) ;
#125130=CARTESIAN_POINT('Ctrl Pts',(0.905822158922318,-3.07467654672654,
1.21201493367489)) ;
#125131=CARTESIAN_POINT('Ctrl Pts',(0.565846680809043,-3.09356407328839,
1.40222551737039)) ;
#125132=CARTESIAN_POINT('Ctrl Pts',(0.383071111602179,-3.10371827157766,
1.46275477782419)) ;
#125133=CARTESIAN_POINT('Ctrl Pts',(-0.0026417638336251,-3.12514676465742,
1.5130356496647)) ;
#125134=CARTESIAN_POINT('Ctrl Pts',(-0.202331067414456,-3.13624061485636,
1.49945057545605)) ;
#125135=CARTESIAN_POINT('Ctrl Pts',(-0.581185047696406,-3.15728805820535,
1.39642875645191)) ;
#125136=CARTESIAN_POINT('Ctrl Pts',(-0.757033408993981,-3.16636065503082,
1.30945917866451)) ;
#125137=CARTESIAN_POINT('Ctrl Pts',(-1.06473075224911,-3.18623331576859,
1.07406282566911)) ;
#125138=CARTESIAN_POINT('Ctrl Pts',(-1.19395549893989,-3.19683653909601,
0.928286909631763)) ;
#125139=CARTESIAN_POINT('Ctrl Pts',(-1.39395362952719,-3.21870607056373,
0.589206208486066)) ;
#125140=CARTESIAN_POINT('Ctrl Pts',(-1.46019955879773,-3.22976372273207,
0.397624329167115)) ;
#125141=CARTESIAN_POINT('Ctrl Pts',(-1.51250754431013,-3.25005028037023,
0.00617617620382795)) ;
#125142=CARTESIAN_POINT('Ctrl Pts',(-1.50060837449239,-3.25909881964487,
-0.189466660143033)) ;
#125143=CARTESIAN_POINT('Ctrl Pts',(-1.40184088383919,-3.28011957356614,
-0.569351388487747)) ;
#125144=CARTESIAN_POINT('Ctrl Pts',(-1.31438594418839,-3.29121473591674,
-0.749467874451868)) ;
#125145=CARTESIAN_POINT('Ctrl Pts',(-1.07900985504578,-3.31266070438634,
-1.05931951010697)) ;
#125146=CARTESIAN_POINT('Ctrl Pts',(-0.935603378011179,-3.32283021821386,
-1.18789311763799)) ;
#125147=CARTESIAN_POINT('Ctrl Pts',(-0.60151270711808,-3.34175786763303,
-1.38840958440627)) ;
#125148=CARTESIAN_POINT('Ctrl Pts',(-0.41241160302782,-3.35208824427622,
-1.45583849950391)) ;
#125149=CARTESIAN_POINT('Ctrl Pts',(-0.144049011394607,-3.36699727714473,
-1.49481720919358)) ;
#125150=CARTESIAN_POINT('Ctrl Pts',(-0.0719924648342288,-3.37100041862031,
-1.5)) ;
#125151=CARTESIAN_POINT('Ctrl Pts',(1.32192589950948E-14,-3.37499999999999,
-1.5)) ;
#125152=CARTESIAN_POINT('Ctrl Pts',(0.,-3.43750000136559,-1.5)) ;
#125153=CARTESIAN_POINT('Ctrl Pts',(-0.0414351247760593,-3.43519804998914,
-1.5)) ;
#125154=CARTESIAN_POINT('Ctrl Pts',(-0.0829168287552058,-3.43289351087919,
-1.49828316721394)) ;
#125155=CARTESIAN_POINT('Ctrl Pts',(-0.322446416719623,-3.41958631154783,
-1.47835938700884)) ;
#125156=CARTESIAN_POINT('Ctrl Pts',(-0.515346390198614,-3.40886964635455,
-1.4226595609534)) ;
#125157=CARTESIAN_POINT('Ctrl Pts',(-0.860329408803675,-3.38970392309872,
-1.24334782196046)) ;
#125158=CARTESIAN_POINT('Ctrl Pts',(-1.01073400139118,-3.38019385287707,
-1.12451242613287)) ;
#125159=CARTESIAN_POINT('Ctrl Pts',(-1.26379037511403,-3.35907435841513,
-0.831654142362913)) ;
#125160=CARTESIAN_POINT('Ctrl Pts',(-1.36198013234628,-3.34802340642958,
-0.658654301400892)) ;
#125161=CARTESIAN_POINT('Ctrl Pts',(-1.48607548799382,-3.32655030240577,
-0.283990702403635)) ;
#125162=CARTESIAN_POINT('Ctrl Pts',(-1.51051733580799,-3.31692760115312,
-0.0859537467911005)) ;
#125163=CARTESIAN_POINT('Ctrl Pts',(-1.4816571571331,-3.29743297384205,
0.302572041010721)) ;
#125164=CARTESIAN_POINT('Ctrl Pts',(-1.43081303000291,-3.28702698592376,
0.489501567854581)) ;
#125165=CARTESIAN_POINT('Ctrl Pts',(-1.25813524563156,-3.26533011978006,
0.840766896875701)) ;
#125166=CARTESIAN_POINT('Ctrl Pts',(-1.13529030741348,-3.25423450246132,
1.00046041397559)) ;
#125167=CARTESIAN_POINT('Ctrl Pts',(-0.840078635521338,-3.23367171450641,
1.25740939753883)) ;
#125168=CARTESIAN_POINT('Ctrl Pts',(-0.672559065071132,-3.22486439386955,
1.35442781593296)) ;
#125169=CARTESIAN_POINT('Ctrl Pts',(-0.30779887117551,-3.20459993865312,
1.48086824581934)) ;
#125170=CARTESIAN_POINT('Ctrl Pts',(-0.113715081646265,-3.1938175059015,
1.50823346071337)) ;
#125171=CARTESIAN_POINT('Ctrl Pts',(0.278712025227951,-3.17201599996404,
1.48722939991194)) ;
#125172=CARTESIAN_POINT('Ctrl Pts',(0.473201068701714,-3.16121105310438,
1.43723140636941)) ;
#125173=CARTESIAN_POINT('Ctrl Pts',(0.82328548612006,-3.14176191880336,
1.26817124058548)) ;
#125174=CARTESIAN_POINT('Ctrl Pts',(0.977057863522894,-3.13254214748269,
1.15387788568608)) ;
#125175=CARTESIAN_POINT('Ctrl Pts',(1.23821659195876,-3.11158827889642,
0.869139967771304)) ;
#125176=CARTESIAN_POINT('Ctrl Pts',(1.34126903660841,-3.10057352373717,
0.699699937605282)) ;
#125177=CARTESIAN_POINT('Ctrl Pts',(1.47729709806211,-3.07890049196363,
0.327770269273075)) ;
#125178=CARTESIAN_POINT('Ctrl Pts',(1.50774033687445,-3.06890015468157,
0.128555803056094)) ;
#125179=CARTESIAN_POINT('Ctrl Pts',(1.48930107103342,-3.04959729792276,
-0.262000625496734)) ;
#125180=CARTESIAN_POINT('Ctrl Pts',(1.44373492322925,-3.03929876374884,
-0.449744010988673)) ;
#125181=CARTESIAN_POINT('Ctrl Pts',(1.28305772881047,-3.0179308183088,-0.80110139540444)) ;
#125182=CARTESIAN_POINT('Ctrl Pts',(1.16819602396499,-3.00705194575476,
-0.96089907910427)) ;
#125183=CARTESIAN_POINT('Ctrl Pts',(0.886799510020267,-2.98654140483531,
-1.22473831358787)) ;
#125184=CARTESIAN_POINT('Ctrl Pts',(0.724038965074748,-2.97772438831419,
-1.32746429229688)) ;
#125185=CARTESIAN_POINT('Ctrl Pts',(0.372142347920373,-2.95817457625006,
-1.46509728046957)) ;
#125186=CARTESIAN_POINT('Ctrl Pts',(0.186817297896326,-2.94787874013761,
-1.5)) ;
#125187=CARTESIAN_POINT('Ctrl Pts',(-4.16333634234434E-16,-2.93750000136559,
-1.5)) ;
#125188=CARTESIAN_POINT('Origin',(0.,-6.,0.)) ;
#125189=CARTESIAN_POINT('',(1.05306898420864E-15,-2.37499999999999,-1.5)) ;
#125190=CARTESIAN_POINT('',(-2.24595708969792E-17,-2.43750000136559,-1.5)) ;
#125191=CARTESIAN_POINT('',(-1.83697019872103E-16,-6.,-1.5)) ;
#125192=CARTESIAN_POINT('Ctrl Pts',(1.83880688453542E-15,-2.37499999999999,
-1.5)) ;
#125193=CARTESIAN_POINT('Ctrl Pts',(0.179045843136507,-2.38494699128535,
-1.5)) ;
#125194=CARTESIAN_POINT('Ctrl Pts',(0.356844193855229,-2.3948246774364,
-1.46794016277328)) ;
#125195=CARTESIAN_POINT('Ctrl Pts',(0.703943741687518,-2.4141079856493,
-1.33827904569682)) ;
#125196=CARTESIAN_POINT('Ctrl Pts',(0.868529861133173,-2.42290477109696,
-1.23781478711461)) ;
#125197=CARTESIAN_POINT('Ctrl Pts',(1.15380320041922,-2.44332561450054,
-0.978078166643146)) ;
#125198=CARTESIAN_POINT('Ctrl Pts',(1.27086028245954,-2.45417091080648,
-0.820245853769252)) ;
#125199=CARTESIAN_POINT('Ctrl Pts',(1.43990537762083,-2.47596007012258,
-0.464964913089586)) ;
#125200=CARTESIAN_POINT('Ctrl Pts',(1.48879898154894,-2.48668768952965,
-0.270224266191242)) ;
#125201=CARTESIAN_POINT('Ctrl Pts',(1.50735577308132,-2.50588727499066,
0.118117855255059)) ;
#125202=CARTESIAN_POINT('Ctrl Pts',(1.48031180593145,-2.51535894825184,
0.307862760530866)) ;
#125203=CARTESIAN_POINT('Ctrl Pts',(1.3545391434805,-2.53645895512261,0.673803287290782)) ;
#125204=CARTESIAN_POINT('Ctrl Pts',(1.25446628635798,-2.5475061069721,0.845636935679458)) ;
#125205=CARTESIAN_POINT('Ctrl Pts',(0.99303044534197,-2.56900349033031,
1.14151160496747)) ;
#125206=CARTESIAN_POINT('Ctrl Pts',(0.833981721521096,-2.57866768213772,
1.26238308549651)) ;
#125207=CARTESIAN_POINT('Ctrl Pts',(0.483487806892448,-2.59813956628375,
1.43285511112529)) ;
#125208=CARTESIAN_POINT('Ctrl Pts',(0.296405157239994,-2.60853304682,1.4828883767912)) ;
#125209=CARTESIAN_POINT('Ctrl Pts',(-0.0939180130779636,-2.63021766739322,
1.51027982196163)) ;
#125210=CARTESIAN_POINT('Ctrl Pts',(-0.29365800396888,-2.64131433355382,
1.48443330920183)) ;
#125211=CARTESIAN_POINT('Ctrl Pts',(-0.664268866896788,-2.66190382593871,
1.35852851474607)) ;
#125212=CARTESIAN_POINT('Ctrl Pts',(-0.832472488380221,-2.67071673287117,
1.26247457376114)) ;
#125213=CARTESIAN_POINT('Ctrl Pts',(-1.12521525458455,-2.69096049698547,
1.01073095284365)) ;
#125214=CARTESIAN_POINT('Ctrl Pts',(-1.24643084741289,-2.70173420805323,
0.856787428527987)) ;
#125215=CARTESIAN_POINT('Ctrl Pts',(-1.42561838823675,-2.72353622496772,
0.50709499141758)) ;
#125216=CARTESIAN_POINT('Ctrl Pts',(-1.48022159937158,-2.73435073531192,
0.313844793563222)) ;
#125217=CARTESIAN_POINT('Ctrl Pts',(-1.51017114759058,-2.75383218337074,
-0.0737781208251271)) ;
#125218=CARTESIAN_POINT('Ctrl Pts',(-1.48872089276062,-2.76302339992767,
-0.264174288743228)) ;
#125219=CARTESIAN_POINT('Ctrl Pts',(-1.37397700269541,-2.78395801818002,
-0.633044742327755)) ;
#125220=CARTESIAN_POINT('Ctrl Pts',(-1.27939778464178,-2.7949680115897,
-0.807277821043497)) ;
#125221=CARTESIAN_POINT('Ctrl Pts',(-1.02627530537409,-2.8166633570728,
-1.11206677747424)) ;
#125222=CARTESIAN_POINT('Ctrl Pts',(-0.869199899582457,-2.82671111668986,
-1.23870531056205)) ;
#125223=CARTESIAN_POINT('Ctrl Pts',(-0.522145877061563,-2.8459918957188,
-1.41915592803456)) ;
#125224=CARTESIAN_POINT('Ctrl Pts',(-0.336999910677903,-2.85627778274012,
-1.4741264970106)) ;
#125225=CARTESIAN_POINT('Ctrl Pts',(-0.0977631271775219,-2.8695687151568,
-1.49761350529533)) ;
#125226=CARTESIAN_POINT('Ctrl Pts',(-0.048852405561043,-2.87228597746883,
-1.5)) ;
#125227=CARTESIAN_POINT('Ctrl Pts',(-1.2605732511172E-14,-2.875,-1.5)) ;
#125228=CARTESIAN_POINT('Ctrl Pts',(0.,-2.93750000136559,-1.5)) ;
#125229=CARTESIAN_POINT('Ctrl Pts',(-0.0132523212698805,-2.93676376129504,
-1.5)) ;
#125230=CARTESIAN_POINT('Ctrl Pts',(-0.026512151688511,-2.93602710404956,
-1.49982437670836)) ;
#125231=CARTESIAN_POINT('Ctrl Pts',(-0.232382246772646,-2.92458987654489,
-1.49436332168044)) ;
#125232=CARTESIAN_POINT('Ctrl Pts',(-0.42223498468532,-2.91404250221641,
-1.45219084965621)) ;
#125233=CARTESIAN_POINT('Ctrl Pts',(-0.77793923996282,-2.89428115470099,
-1.29727969127008)) ;
#125234=CARTESIAN_POINT('Ctrl Pts',(-0.94000408053958,-2.8850748885874,
-1.18512690941558)) ;
#125235=CARTESIAN_POINT('Ctrl Pts',(-1.21389970388962,-2.8638978065848,
-0.903103237471781)) ;
#125236=CARTESIAN_POINT('Ctrl Pts',(-1.32230634146135,-2.85281253025025,
-0.735288696927187)) ;
#125237=CARTESIAN_POINT('Ctrl Pts',(-1.46505521612337,-2.83146796669241,
-0.374066375569203)) ;
#125238=CARTESIAN_POINT('Ctrl Pts',(-1.50065473529158,-2.82142771299859,
-0.185180990127344)) ;
#125239=CARTESIAN_POINT('Ctrl Pts',(-1.4992977711023,-2.80266394994054,
0.204033057725338)) ;
#125240=CARTESIAN_POINT('Ctrl Pts',(-1.45908938348214,-2.79208526701016,
0.400692530060151)) ;
#125241=CARTESIAN_POINT('Ctrl Pts',(-1.305666754252,-2.77035162712593,0.763839155929079)) ;
#125242=CARTESIAN_POINT('Ctrl Pts',(-1.19510987201921,-2.75941481549434,
0.927326471235875)) ;
#125243=CARTESIAN_POINT('Ctrl Pts',(-0.921200286387028,-2.73873538151063,
1.19899866221631)) ;
#125244=CARTESIAN_POINT('Ctrl Pts',(-0.76186745976206,-2.72982597135238,
1.30604686821552)) ;
#125245=CARTESIAN_POINT('Ctrl Pts',(-0.401830477127252,-2.70982391676155,
1.45907902690513)) ;
#125246=CARTESIAN_POINT('Ctrl Pts',(-0.202995714400276,-2.6987775410545,
1.49971794259337)) ;
#125247=CARTESIAN_POINT('Ctrl Pts',(0.191096578722603,-2.67688352476989,
1.50026836417804)) ;
#125248=CARTESIAN_POINT('Ctrl Pts',(0.382553545209961,-2.6662470266317,
1.46321266530721)) ;
#125249=CARTESIAN_POINT('Ctrl Pts',(0.741491518165052,-2.6463060281342,
1.31824794173905)) ;
#125250=CARTESIAN_POINT('Ctrl Pts',(0.905463088608233,-2.63730316853214,
1.21149858735916)) ;
#125251=CARTESIAN_POINT('Ctrl Pts',(1.18701578749506,-2.61633707960545,
0.938281138768189)) ;
#125252=CARTESIAN_POINT('Ctrl Pts',(1.30059020178559,-2.60523969723543,
0.773198596281036)) ;
#125253=CARTESIAN_POINT('Ctrl Pts',(1.45396456412132,-2.58375897476809,
0.415280893301883)) ;
#125254=CARTESIAN_POINT('Ctrl Pts',(1.49498684495197,-2.57355865072957,
0.226955364321571)) ;
#125255=CARTESIAN_POINT('Ctrl Pts',(1.50433565895458,-2.55454999214157,
-0.162734644895059)) ;
#125256=CARTESIAN_POINT('Ctrl Pts',(1.46956061091959,-2.54431087635249,
-0.360479674535448)) ;
#125257=CARTESIAN_POINT('Ctrl Pts',(1.32589085798636,-2.52262288504127,
-0.728308338386614)) ;
#125258=CARTESIAN_POINT('Ctrl Pts',(1.21947671138053,-2.51163959036419,
-0.895153595180616)) ;
#125259=CARTESIAN_POINT('Ctrl Pts',(0.952647844145463,-2.49080569364162,
-1.17412428857262)) ;
#125260=CARTESIAN_POINT('Ctrl Pts',(0.79644403135156,-2.48174689199624,
-1.28521198093932)) ;
#125261=CARTESIAN_POINT('Ctrl Pts',(0.442771250326625,-2.46209840416152,
-1.44689800637849)) ;
#125262=CARTESIAN_POINT('Ctrl Pts',(0.247250914219815,-2.45123616326669,
-1.49278504712828)) ;
#125263=CARTESIAN_POINT('Ctrl Pts',(0.0323322730512658,-2.43929623875733,
-1.49973882485724)) ;
#125264=CARTESIAN_POINT('Ctrl Pts',(0.0161609579953818,-2.43839783236533,
-1.5)) ;
#125265=CARTESIAN_POINT('Ctrl Pts',(0.,-2.43750000136559,-1.5)) ;
#125266=CARTESIAN_POINT('Origin',(0.,-6.,0.)) ;
#125267=CARTESIAN_POINT('',(-1.23676600408074E-15,-1.87499999999999,-1.5)) ;
#125268=CARTESIAN_POINT('',(2.06788221765507E-15,-1.93750000136559,-1.5)) ;
#125269=CARTESIAN_POINT('',(-1.83697019872103E-16,-6.,-1.5)) ;
#125270=CARTESIAN_POINT('Ctrl Pts',(2.60282034651221E-16,-1.87499999999999,
-1.5)) ;
#125271=CARTESIAN_POINT('Ctrl Pts',(0.00943735868268793,-1.87552429770459,
-1.5)) ;
#125272=CARTESIAN_POINT('Ctrl Pts',(0.0188785514875759,-1.87604880841598,
-1.49991093644605)) ;
#125273=CARTESIAN_POINT('Ctrl Pts',(0.22714652682835,-1.88761925149046,
-1.49597781079793)) ;
#125274=CARTESIAN_POINT('Ctrl Pts',(0.4232774234807,-1.89851541241559,-1.45272168687975)) ;
#125275=CARTESIAN_POINT('Ctrl Pts',(0.779208648772136,-1.91828936937623,
-1.29575149131839)) ;
#125276=CARTESIAN_POINT('Ctrl Pts',(0.93697217883324,-1.92726573334301,
-1.18668907950213)) ;
#125277=CARTESIAN_POINT('Ctrl Pts',(1.20736056247296,-1.94802262290301,
-0.911374037682096)) ;
#125278=CARTESIAN_POINT('Ctrl Pts',(1.31586542221273,-1.95898355504511,
-0.746200651240154)) ;
#125279=CARTESIAN_POINT('Ctrl Pts',(1.4644642889903,-1.98069920720196,-0.380642892713603)) ;
#125280=CARTESIAN_POINT('Ctrl Pts',(1.50194695578602,-1.99112086962977,
-0.183425183692144)) ;
#125281=CARTESIAN_POINT('Ctrl Pts',(1.49797825778615,-2.00996969178462,
0.206048899069629)) ;
#125282=CARTESIAN_POINT('Ctrl Pts',(1.45965998564815,-2.02010908144715,
0.394669090974854)) ;
#125283=CARTESIAN_POINT('Ctrl Pts',(1.31163447008062,-2.04152055546697,
0.754235650122164)) ;
#125284=CARTESIAN_POINT('Ctrl Pts',(1.20064793304481,-2.0526130092772,0.920709866047377)) ;
#125285=CARTESIAN_POINT('Ctrl Pts',(0.92292434835193,-2.07368596213456,
1.19835917983805)) ;
#125286=CARTESIAN_POINT('Ctrl Pts',(0.759912420907417,-2.08278264328292,
1.30781507008685)) ;
#125287=CARTESIAN_POINT('Ctrl Pts',(0.40259446922281,-2.10263364059874,
1.4577915896283)) ;
#125288=CARTESIAN_POINT('Ctrl Pts',(0.211929265373631,-2.11322615192369,
1.49743386092166)) ;
#125289=CARTESIAN_POINT('Ctrl Pts',(-0.181574388459856,-2.13508746602555,
1.50242238157228)) ;
#125290=CARTESIAN_POINT('Ctrl Pts',(-0.380671142079628,-2.1461483967822,
1.46470086422455)) ;
#125291=CARTESIAN_POINT('Ctrl Pts',(-0.742849037099933,-2.16626939094999,
1.31699025508058)) ;
#125292=CARTESIAN_POINT('Ctrl Pts',(-0.903904054165086,-2.17512331637634,
1.21212648927073)) ;
#125293=CARTESIAN_POINT('Ctrl Pts',(-1.18160979654635,-2.19571782871237,
0.944411073712693)) ;
#125294=CARTESIAN_POINT('Ctrl Pts',(-1.29435969760203,-2.20662639734714,
0.782776918078987)) ;
#125295=CARTESIAN_POINT('Ctrl Pts',(-1.45302295344634,-2.2283833369147,
0.422171694572619)) ;
#125296=CARTESIAN_POINT('Ctrl Pts',(-1.49613045578213,-2.23901395315421,
0.226106613339065)) ;
#125297=CARTESIAN_POINT('Ctrl Pts',(-1.50321487640017,-2.25792417813516,
-0.162844839904798)) ;
#125298=CARTESIAN_POINT('Ctrl Pts',(-1.47048115626658,-2.26775558478375,
-0.352000187186925)) ;
#125299=CARTESIAN_POINT('Ctrl Pts',(-1.33342945165836,-2.2890194806551,
-0.714835124830947)) ;
#125300=CARTESIAN_POINT('Ctrl Pts',(-1.22780151418331,-2.30009454820616,
-0.884041763044062)) ;
#125301=CARTESIAN_POINT('Ctrl Pts',(-0.958042844808662,-2.32138113354333,
-1.17072989054784)) ;
#125302=CARTESIAN_POINT('Ctrl Pts',(-0.796989535015222,-2.33072280361027,
-1.2857875225238)) ;
#125303=CARTESIAN_POINT('Ctrl Pts',(-0.443022474300268,-2.35038764031665,
-1.44594879262274)) ;
#125304=CARTESIAN_POINT('Ctrl Pts',(-0.254069427816286,-2.36088503178798,
-1.49079413572083)) ;
#125305=CARTESIAN_POINT('Ctrl Pts',(-0.0412129187210752,-2.37271039340438,
-1.49957571771944)) ;
#125306=CARTESIAN_POINT('Ctrl Pts',(-0.0205982039601356,-2.37385565533554,
-1.5)) ;
#125307=CARTESIAN_POINT('Ctrl Pts',(2.6028203465122E-16,-2.37499999999999,
-1.5)) ;
#125308=CARTESIAN_POINT('Ctrl Pts',(-1.07552855510562E-15,-2.43750000136559,
-1.5)) ;
#125309=CARTESIAN_POINT('Ctrl Pts',(-0.177332442740351,-2.42764819899113,
-1.5)) ;
#125310=CARTESIAN_POINT('Ctrl Pts',(-0.353417850306997,-2.41786567634853,
-1.46855134717232)) ;
#125311=CARTESIAN_POINT('Ctrl Pts',(-0.700665072932742,-2.39857416398043,
-1.34020877878796)) ;
#125312=CARTESIAN_POINT('Ctrl Pts',(-0.866743242519118,-2.38971601567301,
-1.23929375986335)) ;
#125313=CARTESIAN_POINT('Ctrl Pts',(-1.15650631385966,-2.36898820306878,
-0.975769052379438)) ;
#125314=CARTESIAN_POINT('Ctrl Pts',(-1.27564803794744,-2.35788815355817,
-0.813845362226324)) ;
#125315=CARTESIAN_POINT('Ctrl Pts',(-1.44058755834756,-2.33627150333408,
-0.459779600998612)) ;
#125316=CARTESIAN_POINT('Ctrl Pts',(-1.4874822923766,-2.32594524830586,
-0.272227107984242)) ;
#125317=CARTESIAN_POINT('Ctrl Pts',(-1.5085508736479,-2.30659366029616,
0.117824144626538)) ;
#125318=CARTESIAN_POINT('Ctrl Pts',(-1.47963309169109,-2.29669516685316,
0.316738476574083)) ;
#125319=CARTESIAN_POINT('Ctrl Pts',(-1.34662537643692,-2.27507190351172,
0.689377525161628)) ;
#125320=CARTESIAN_POINT('Ctrl Pts',(-1.24479148771335,-2.26404706697388,
0.859730626438732)) ;
#125321=CARTESIAN_POINT('Ctrl Pts',(-0.985673414919529,-2.24305083706711,
1.14652718095046)) ;
#125322=CARTESIAN_POINT('Ctrl Pts',(-0.832760732880199,-2.2337644865256,
1.26196855215552)) ;
#125323=CARTESIAN_POINT('Ctrl Pts',(-0.483964356688177,-2.21438691007049,
1.43364193376676)) ;
#125324=CARTESIAN_POINT('Ctrl Pts',(-0.289863219534461,-2.20360351356195,
1.48509519379718)) ;
#125325=CARTESIAN_POINT('Ctrl Pts',(0.102527341581848,-2.18180403794437,
1.50905337356658)) ;
#125326=CARTESIAN_POINT('Ctrl Pts',(0.296950144442835,-2.17100277111876,
1.48309999427456)) ;
#125327=CARTESIAN_POINT('Ctrl Pts',(0.662529120150319,-2.1506928280239,
1.35932974810785)) ;
#125328=CARTESIAN_POINT('Ctrl Pts',(0.83056065201908,-2.14189443954733,
1.26368142146705)) ;
#125329=CARTESIAN_POINT('Ctrl Pts',(1.12768045373333,-2.12139066244948,
1.00906061480182)) ;
#125330=CARTESIAN_POINT('Ctrl Pts',(1.25182239011894,-2.11029780742779,
0.850173333209126)) ;
#125331=CARTESIAN_POINT('Ctrl Pts',(1.42721924685902,-2.08857483450314,
0.499935242099737)) ;
#125332=CARTESIAN_POINT('Ctrl Pts',(1.47945500711303,-2.07814170737608,
0.313245097152927)) ;
#125333=CARTESIAN_POINT('Ctrl Pts',(1.511052979967,-2.05859730310795,-0.0747346190667385)) ;
#125334=CARTESIAN_POINT('Ctrl Pts',(1.48816846050364,-2.04906221844655,
-0.272468130568953)) ;
#125335=CARTESIAN_POINT('Ctrl Pts',(1.36719082913346,-2.02764278422735,
-0.647816242575988)) ;
#125336=CARTESIAN_POINT('Ctrl Pts',(1.2702926922646,-2.01658398592398,-0.821724883555877)) ;
#125337=CARTESIAN_POINT('Ctrl Pts',(1.01937149866044,-1.99542199406449,
-1.11669920596306)) ;
#125338=CARTESIAN_POINT('Ctrl Pts',(0.869834738526956,-1.98582415350598,
-1.23672475538724)) ;
#125339=CARTESIAN_POINT('Ctrl Pts',(0.526189893171804,-1.96673277320847,
-1.4186835775582)) ;
#125340=CARTESIAN_POINT('Ctrl Pts',(0.333729565204767,-1.95604053276585,
-1.47585193693545)) ;
#125341=CARTESIAN_POINT('Ctrl Pts',(0.0905495303401054,-1.94253053082893,
-1.49795258490765)) ;
#125342=CARTESIAN_POINT('Ctrl Pts',(0.0452488974255713,-1.94001382900035,
-1.5)) ;
#125343=CARTESIAN_POINT('Ctrl Pts',(0.,-1.93750000136559,-1.5)) ;
#125344=CARTESIAN_POINT('Origin',(0.,-6.,0.)) ;
#125345=CARTESIAN_POINT('',(-1.83697019872103E-16,-0.1,-1.5)) ;
#125346=CARTESIAN_POINT('Origin',(0.,-0.1,0.)) ;
#125347=CARTESIAN_POINT('',(1.27966723825811E-15,-0.93750000136559,-1.5)) ;
#125348=CARTESIAN_POINT('',(-1.83697019872103E-16,-6.,-1.5)) ;
#125349=CARTESIAN_POINT('',(1.48723526368499,-0.552750382528326,-0.19527229821924)) ;
#125350=CARTESIAN_POINT('Ctrl Pts',(0.,-0.93750000136559,-1.5)) ;
#125351=CARTESIAN_POINT('Ctrl Pts',(-0.0924142321550466,-0.932365877356976,
-1.5)) ;
#125352=CARTESIAN_POINT('Ctrl Pts',(-0.184851853456529,-0.927230453951329,
-1.49145967026687)) ;
#125353=CARTESIAN_POINT('Ctrl Pts',(-0.462932371399564,-0.911781536287827,
-1.43938052160168)) ;
#125354=CARTESIAN_POINT('Ctrl Pts',(-0.641347933989665,-0.902228062825542,
-1.36921973430852)) ;
#125355=CARTESIAN_POINT('Ctrl Pts',(-0.969943538414926,-0.883099606137119,
-1.16135698872124)) ;
#125356=CARTESIAN_POINT('Ctrl Pts',(-1.11516010244463,-0.872395120488618,
-1.02270925490941)) ;
#125357=CARTESIAN_POINT('Ctrl Pts',(-1.3407638224346,-0.850612138321202,
-0.700210841123837)) ;
#125358=CARTESIAN_POINT('Ctrl Pts',(-1.42027434193999,-0.839750349397203,
-0.52035821763424)) ;
#125359=CARTESIAN_POINT('Ctrl Pts',(-1.50522706343029,-0.819286071047164,
-0.144063656145068)) ;
#125360=CARTESIAN_POINT('Ctrl Pts',(-1.51132705318559,-0.810481931552609,
0.0484844705972081)) ;
#125361=CARTESIAN_POINT('Ctrl Pts',(-1.44951895516163,-0.790182777922516,
0.434709533820591)) ;
#125362=CARTESIAN_POINT('Ctrl Pts',(-1.37863155578292,-0.779104061815861,
0.624049464859449)) ;
#125363=CARTESIAN_POINT('Ctrl Pts',(-1.17080022717307,-0.75730064673869,
0.957233463646603)) ;
#125364=CARTESIAN_POINT('Ctrl Pts',(-1.03838420938941,-0.746778825997023,
1.09947497748658)) ;
#125365=CARTESIAN_POINT('Ctrl Pts',(-0.724474918368461,-0.727067156923346,
1.32793871186564)) ;
#125366=CARTESIAN_POINT('Ctrl Pts',(-0.545281412466567,-0.717793413169278,
1.41101535151924)) ;
#125367=CARTESIAN_POINT('Ctrl Pts',(-0.163073280254602,-0.696559628046391,
1.50415834013272)) ;
#125368=CARTESIAN_POINT('Ctrl Pts',(0.0363728332714122,-0.685479288406057,
1.51253380685678)) ;
#125369=CARTESIAN_POINT('Ctrl Pts',(0.419829625717041,-0.664176133270189,
1.45258543441048)) ;
#125370=CARTESIAN_POINT('Ctrl Pts',(0.600589014989293,-0.654245791110056,
1.38762525630755)) ;
#125371=CARTESIAN_POINT('Ctrl Pts',(0.935392040807353,-0.635406495702389,
1.18935647149059)) ;
#125372=CARTESIAN_POINT('Ctrl Pts',(1.08459357960647,-0.62480079948512,
1.05506276370435)) ;
#125373=CARTESIAN_POINT('Ctrl Pts',(1.31990170521924,-0.603054571176904,
0.738931105735517)) ;
#125374=CARTESIAN_POINT('Ctrl Pts',(1.40481888017356,-0.592132013847489,
0.56093696863664)) ;
#125375=CARTESIAN_POINT('Ctrl Pts',(1.50056674105296,-0.571460167677666,
0.186560767661118)) ;
#125376=CARTESIAN_POINT('Ctrl Pts',(1.51210623124261,-0.562554840242503,
-0.00584973121425299)) ;
#125377=CARTESIAN_POINT('Ctrl Pts',(1.48723526368499,-0.552750382528326,
-0.19527229821924)) ;
#125378=CARTESIAN_POINT('',(0.903681962956226,-0.694267812214528,-1.19722968131749)) ;
#125379=CARTESIAN_POINT('Origin',(0.,-1.40417355919753,0.)) ;
#125380=CARTESIAN_POINT('',(0.903681962086507,-0.819267341061323,-1.19722968197397)) ;
#125381=CARTESIAN_POINT('',(0.903681962956226,-0.694267812214528,-1.19722968131749)) ;
#125382=CARTESIAN_POINT('',(1.42658067231545,-0.975658586206326,-0.463538116421942)) ;
#125383=CARTESIAN_POINT('Origin',(0.,-0.109621223236985,0.)) ;
#125384=CARTESIAN_POINT('',(-9.18485099360515E-17,-1.37499999999999,-1.5)) ;
#125385=CARTESIAN_POINT('Ctrl Pts',(1.42658067231545,-0.975658586206326,
-0.463538116421941)) ;
#125386=CARTESIAN_POINT('Ctrl Pts',(1.4608676911025,-0.981687904878683,
-0.35801670064177)) ;
#125387=CARTESIAN_POINT('Ctrl Pts',(1.4833430518337,-0.987556547803326,
-0.249015403606839)) ;
#125388=CARTESIAN_POINT('Ctrl Pts',(1.50354576305376,-0.998598705815113,
-0.0311724999487236)) ;
#125389=CARTESIAN_POINT('Ctrl Pts',(1.50190176982991,-1.00364732798507,
0.0769062759071393)) ;
#125390=CARTESIAN_POINT('Ctrl Pts',(1.46503210262907,-1.01903086279124,
0.375360330235355)) ;
#125391=CARTESIAN_POINT('Ctrl Pts',(1.40467081292517,-1.02961241555355,
0.560444167463701)) ;
#125392=CARTESIAN_POINT('Ctrl Pts',(1.21347769961073,-1.05146516319492,
0.90425960242237)) ;
#125393=CARTESIAN_POINT('Ctrl Pts',(1.08184553656645,-1.06252928019626,
1.0582250911012)) ;
#125394=CARTESIAN_POINT('Ctrl Pts',(0.773696965752526,-1.08267888640319,
1.29911713122624)) ;
#125395=CARTESIAN_POINT('Ctrl Pts',(0.602602377832728,-1.09152209012042,
1.3867903141585)) ;
#125396=CARTESIAN_POINT('Ctrl Pts',(0.232273153510163,-1.11209593591611,
1.4947030359203)) ;
#125397=CARTESIAN_POINT('Ctrl Pts',(0.0360475909930078,-1.12299735605596,
1.51221063712791)) ;
#125398=CARTESIAN_POINT('Ctrl Pts',(-0.355665576846667,-1.14475919871371,
1.4707170273039)) ;
#125399=CARTESIAN_POINT('Ctrl Pts',(-0.547235950104445,-1.15540199722803,
1.41069664698689)) ;
#125400=CARTESIAN_POINT('Ctrl Pts',(-0.888252485248476,-1.17434736029159,
1.22358660666486)) ;
#125401=CARTESIAN_POINT('Ctrl Pts',(-1.0361018207849,-1.18413130376333,
1.10122340347657)) ;
#125402=CARTESIAN_POINT('Ctrl Pts',(-1.28281560741993,-1.20537561709001,
0.802108913958369)) ;
#125403=CARTESIAN_POINT('Ctrl Pts',(-1.37715772840634,-1.2164478442942,
0.626445442058699)) ;
#125404=CARTESIAN_POINT('Ctrl Pts',(-1.49202537596067,-1.23776042435012,
0.249790651328553)) ;
#125405=CARTESIAN_POINT('Ctrl Pts',(-1.51186968215624,-1.24713737546132,
0.0526455695399674)) ;
#125406=CARTESIAN_POINT('Ctrl Pts',(-1.47488723137769,-1.26677894559483,
-0.334244971487723)) ;
#125407=CARTESIAN_POINT('Ctrl Pts',(-1.41990947355275,-1.2772640810985,
-0.520432997207323)) ;
#125408=CARTESIAN_POINT('Ctrl Pts',(-1.23916679121819,-1.29903518512036,
-0.868585060540103)) ;
#125409=CARTESIAN_POINT('Ctrl Pts',(-1.11248140632144,-1.31012075688599,
-1.02585250181586)) ;
#125410=CARTESIAN_POINT('Ctrl Pts',(-0.811619236320399,-1.33050687516637,
-1.27586715854565)) ;
#125411=CARTESIAN_POINT('Ctrl Pts',(-0.642569451667573,-1.33930169712959,
-1.36882027675838)) ;
#125412=CARTESIAN_POINT('Ctrl Pts',(-0.311549635183878,-1.35769168693423,
-1.47562252873181)) ;
#125413=CARTESIAN_POINT('Ctrl Pts',(-0.156126656755279,-1.36632629684692,
-1.5)) ;
#125414=CARTESIAN_POINT('Ctrl Pts',(5.89805981832114E-16,-1.37499999999999,
-1.5)) ;
#125415=CARTESIAN_POINT('',(-2.10412774206915E-15,-1.43750000136559,-1.5)) ;
#125416=CARTESIAN_POINT('',(-1.83697019872103E-16,-6.,-1.5)) ;
#125417=CARTESIAN_POINT('Ctrl Pts',(-1.45716771982052E-15,-1.43750000136559,
-1.5)) ;
#125418=CARTESIAN_POINT('Ctrl Pts',(-0.12139289337904,-1.43075595173342,
-1.5)) ;
#125419=CARTESIAN_POINT('Ctrl Pts',(-0.242615485235266,-1.42402136329696,
-1.48526320021271)) ;
#125420=CARTESIAN_POINT('Ctrl Pts',(-0.54542560532699,-1.40719857884742,
-1.41018650153551)) ;
#125421=CARTESIAN_POINT('Ctrl Pts',(-0.719475265230306,-1.39816291148787,
-1.32983398614367)) ;
#125422=CARTESIAN_POINT('Ctrl Pts',(-1.03556294373952,-1.37848139126207,
-1.1032545764031)) ;
#125423=CARTESIAN_POINT('Ctrl Pts',(-1.17254730770333,-1.36761005677763,
-0.956386091734899)) ;
#125424=CARTESIAN_POINT('Ctrl Pts',(-1.37853603313159,-1.34581062140582,
-0.622220982127438)) ;
#125425=CARTESIAN_POINT('Ctrl Pts',(-1.44729330200646,-1.33509397144994,
-0.439176623295063)) ;
#125426=CARTESIAN_POINT('Ctrl Pts',(-1.51121609450788,-1.31498083622332,
-0.0580387994088512)) ;
#125427=CARTESIAN_POINT('Ctrl Pts',(-1.50617017426866,-1.30611041853233,
0.136367337051198)) ;
#125428=CARTESIAN_POINT('Ctrl Pts',(-1.42141652159494,-1.28535520160221,
0.518823875806305)) ;
#125429=CARTESIAN_POINT('Ctrl Pts',(-1.34012610682817,-1.27425489967523,
0.702606275960677)) ;
#125430=CARTESIAN_POINT('Ctrl Pts',(-1.11491907204454,-1.25265264228599,
1.02157742208114)) ;
#125431=CARTESIAN_POINT('Ctrl Pts',(-0.97552501409157,-1.24234020400036,
1.15543822992624)) ;
#125432=CARTESIAN_POINT('Ctrl Pts',(-0.647387975472766,-1.22301296441911,
1.36769735344609)) ;
#125433=CARTESIAN_POINT('Ctrl Pts',(-0.460153323374986,-1.21306407488642,
1.44152590664843)) ;
#125434=CARTESIAN_POINT('Ctrl Pts',(-0.0704853868697509,-1.19141585619168,
1.51117296929148)) ;
#125435=CARTESIAN_POINT('Ctrl Pts',(0.127872336502056,-1.18039598267102,
1.50740248439617)) ;
#125436=CARTESIAN_POINT('Ctrl Pts',(0.505423896210884,-1.15942089602053,
1.42499909293535)) ;
#125437=CARTESIAN_POINT('Ctrl Pts',(0.681572805914866,-1.1501684229538,
1.34963476410479)) ;
#125438=CARTESIAN_POINT('Ctrl Pts',(1.0038364982207,-1.13075505293512,1.13219447498585)) ;
#125439=CARTESIAN_POINT('Ctrl Pts',(1.14491523340415,-1.11996081308417,
0.989292258509651)) ;
#125440=CARTESIAN_POINT('Ctrl Pts',(1.3605913200847,-1.09816016784024,0.660695002809255)) ;
#125441=CARTESIAN_POINT('Ctrl Pts',(1.43463121008879,-1.08736823961763,
0.479135937315464)) ;
#125442=CARTESIAN_POINT('Ctrl Pts',(1.50887308707389,-1.06708098933289,
0.100336926109472)) ;
#125443=CARTESIAN_POINT('Ctrl Pts',(1.50933516496826,-1.05827872850654,
-0.0931271687809125)) ;
#125444=CARTESIAN_POINT('Ctrl Pts',(1.43590454263757,-1.03774545194468,
-0.477508118223692)) ;
#125445=CARTESIAN_POINT('Ctrl Pts',(1.35970219382423,-1.02665114013334,
-0.664103612410434)) ;
#125446=CARTESIAN_POINT('Ctrl Pts',(1.14296119693593,-1.00494105320597,
-0.990203822651857)) ;
#125447=CARTESIAN_POINT('Ctrl Pts',(1.00694889425996,-0.994521405798722,
-1.12824538756443)) ;
#125448=CARTESIAN_POINT('Ctrl Pts',(0.685828290440808,-0.975001799998438,
-1.34855370838484)) ;
#125449=CARTESIAN_POINT('Ctrl Pts',(0.502625072513882,-0.965423616505241,
-1.4270054983915)) ;
#125450=CARTESIAN_POINT('Ctrl Pts',(0.207451669629485,-0.949025094122774,
-1.4892377999239)) ;
#125451=CARTESIAN_POINT('Ctrl Pts',(0.103740571639932,-0.943263366456697,
-1.5)) ;
#125452=CARTESIAN_POINT('Ctrl Pts',(-3.81639164714898E-16,-0.93750000136559,
-1.5)) ;
#125453=CARTESIAN_POINT('Origin',(0.,-6.,0.)) ;
#125454=CARTESIAN_POINT('Ctrl Pts',(2.60282034651221E-16,-1.37499999999999,
-1.5)) ;
#125455=CARTESIAN_POINT('Ctrl Pts',(0.0378880627307306,-1.37710489237392,
-1.5)) ;
#125456=CARTESIAN_POINT('Ctrl Pts',(0.0758175659488453,-1.37921208699716,
-1.49856452262518)) ;
#125457=CARTESIAN_POINT('Ctrl Pts',(0.31193570823378,-1.39232976156855,
-1.48061396356261)) ;
#125458=CARTESIAN_POINT('Ctrl Pts',(0.505234227970466,-1.40306856822058,
-1.42628306779644)) ;
#125459=CARTESIAN_POINT('Ctrl Pts',(0.851455565955026,-1.4223030869975,
-1.24943605696842)) ;
#125460=CARTESIAN_POINT('Ctrl Pts',(1.002668770544,-1.43173619321328,-1.13170226086917)) ;
#125461=CARTESIAN_POINT('Ctrl Pts',(1.25769711838986,-1.45281601037343,
-0.840807174121323)) ;
#125462=CARTESIAN_POINT('Ctrl Pts',(1.35707620689297,-1.46385909327745,
-0.66865754967684)) ;
#125463=CARTESIAN_POINT('Ctrl Pts',(1.48406103596784,-1.48538141381695,
-0.29463924287184)) ;
#125464=CARTESIAN_POINT('Ctrl Pts',(1.50995001557063,-1.49508944413126,
-0.0963193429286017)) ;
#125465=CARTESIAN_POINT('Ctrl Pts',(1.48362149567478,-1.51453781872515,
0.292706754077122)) ;
#125466=CARTESIAN_POINT('Ctrl Pts',(1.43406250307638,-1.5249183011972,0.479848132943688)) ;
#125467=CARTESIAN_POINT('Ctrl Pts',(1.26389924289045,-1.54659005786061,
0.832043332432613)) ;
#125468=CARTESIAN_POINT('Ctrl Pts',(1.14225570304284,-1.55768766952758,
0.992471928954704)) ;
#125469=CARTESIAN_POINT('Ctrl Pts',(0.84881104050339,-1.5783045798591,1.25156600831668)) ;
#125470=CARTESIAN_POINT('Ctrl Pts',(0.681763120312136,-1.58712427109378,
1.34985039084804)) ;
#125471=CARTESIAN_POINT('Ctrl Pts',(0.317759579117409,-1.60734669004904,
1.47874613221529)) ;
#125472=CARTESIAN_POINT('Ctrl Pts',(0.123996398982104,-1.61811131116766,
1.50740639143056)) ;
#125473=CARTESIAN_POINT('Ctrl Pts',(-0.268444572010862,-1.63991358733394,
1.48911788802839)) ;
#125474=CARTESIAN_POINT('Ctrl Pts',(-0.463280400432789,-1.65073780002404,
1.44046068521351)) ;
#125475=CARTESIAN_POINT('Ctrl Pts',(-0.814543246749689,-1.67025240259721,
1.2738066884214)) ;
#125476=CARTESIAN_POINT('Ctrl Pts',(-0.969108063961199,-1.67941530512131,
1.16056473101709)) ;
#125477=CARTESIAN_POINT('Ctrl Pts',(-1.23213115359432,-1.70033009362367,
0.877715466832144)) ;
#125478=CARTESIAN_POINT('Ctrl Pts',(-1.33629297016389,-1.71133506582633,
0.709119267777291)) ;
#125479=CARTESIAN_POINT('Ctrl Pts',(-1.47508909334509,-1.73305320093322,
0.337850285448988)) ;
#125480=CARTESIAN_POINT('Ctrl Pts',(-1.5069343887875,-1.74315054142095,
0.138359751926198)) ;
#125481=CARTESIAN_POINT('Ctrl Pts',(-1.49090003004465,-1.76240862090636,
-0.252654472236755)) ;
#125482=CARTESIAN_POINT('Ctrl Pts',(-1.44654705011602,-1.77268144862352,
-0.440563981857862)) ;
#125483=CARTESIAN_POINT('Ctrl Pts',(-1.28660460880766,-1.79424170245274,
-0.796342630989032)) ;
#125484=CARTESIAN_POINT('Ctrl Pts',(-1.16986364904193,-1.8053419518461,
-0.959656557554787)) ;
#125485=CARTESIAN_POINT('Ctrl Pts',(-0.883637371833339,-1.8261739373672,
-1.22738842750026)) ;
#125486=CARTESIAN_POINT('Ctrl Pts',(-0.718475544917168,-1.83508469194905,
-1.33082202979742)) ;
#125487=CARTESIAN_POINT('Ctrl Pts',(-0.366370874060449,-1.8546460625522,
-1.46617447464151)) ;
#125488=CARTESIAN_POINT('Ctrl Pts',(-0.183913488692333,-1.86478258396153,
-1.5)) ;
#125489=CARTESIAN_POINT('Ctrl Pts',(3.81639164714898E-16,-1.87499999999999,
-1.5)) ;
#125490=CARTESIAN_POINT('Ctrl Pts',(-5.20417042793042E-16,-1.93750000136559,
-1.5)) ;
#125491=CARTESIAN_POINT('Ctrl Pts',(-0.148963326007169,-1.92922426103186,
-1.5)) ;
#125492=CARTESIAN_POINT('Ctrl Pts',(-0.297365951084213,-1.9209796707498,
-1.4778082396457)) ;
#125493=CARTESIAN_POINT('Ctrl Pts',(-0.622721506224344,-1.9029043621309,
-1.37791446022743)) ;
#125494=CARTESIAN_POINT('Ctrl Pts',(-0.792785345987669,-1.89409462925514,
-1.28760192268381)) ;
#125495=CARTESIAN_POINT('Ctrl Pts',(-1.09729928647212,-1.87382581947286,
-1.04213382797214)) ;
#125496=CARTESIAN_POINT('Ctrl Pts',(-1.22646524414687,-1.86274978204871,
-0.886496713623897)) ;
#125497=CARTESIAN_POINT('Ctrl Pts',(-1.4124393734564,-1.8409357283315,-0.540472334956)) ;
#125498=CARTESIAN_POINT('Ctrl Pts',(-1.4701082237838,-1.83040144918074,
-0.354816580693619)) ;
#125499=CARTESIAN_POINT('Ctrl Pts',(-1.51236437049839,-1.81066565131077,
0.0309876772900098)) ;
#125500=CARTESIAN_POINT('Ctrl Pts',(-1.49546953995707,-1.80142527481105,
0.227568206543377)) ;
#125501=CARTESIAN_POINT('Ctrl Pts',(-1.38655761046561,-1.78021894123352,
0.605453241115908)) ;
#125502=CARTESIAN_POINT('Ctrl Pts',(-1.29473792765022,-1.76913611908959,
0.782793255060013)) ;
#125503=CARTESIAN_POINT('Ctrl Pts',(-1.05215553348107,-1.74781282097243,
1.08593467317216)) ;
#125504=CARTESIAN_POINT('Ctrl Pts',(-0.905935169714077,-1.73782973301637,
1.21058411696564)) ;
#125505=CARTESIAN_POINT('Ctrl Pts',(-0.567487526947019,-1.71902708619598,
1.40267001389958)) ;
#125506=CARTESIAN_POINT('Ctrl Pts',(-0.376819826414949,-1.70843443616642,
1.46543693014733)) ;
#125507=CARTESIAN_POINT('Ctrl Pts',(0.0145050608199446,-1.68669416465337,
1.51260589749027)) ;
#125508=CARTESIAN_POINT('Ctrl Pts',(0.211237065013851,-1.67576460886482,
1.49785589403808)) ;
#125509=CARTESIAN_POINT('Ctrl Pts',(0.583064477857225,-1.65510753037352,
1.39508568987848)) ;
#125510=CARTESIAN_POINT('Ctrl Pts',(0.755163912351607,-1.64621452491384,
1.30994238169818)) ;
#125511=CARTESIAN_POINT('Ctrl Pts',(1.06678098124075,-1.62618094467741,
1.07346443438125)) ;
#125512=CARTESIAN_POINT('Ctrl Pts',(1.20076273752401,-1.61513050794521,
0.921139823045825)) ;
#125513=CARTESIAN_POINT('Ctrl Pts',(1.39694502659761,-1.59324470839863,
0.57951791910547)) ;
#125514=CARTESIAN_POINT('Ctrl Pts',(1.45988754717958,-1.58261962593753,
0.395019608420067)) ;
#125515=CARTESIAN_POINT('Ctrl Pts',(1.51245624265528,-1.56270225690715,
0.0113954175393681)) ;
#125516=CARTESIAN_POINT('Ctrl Pts',(1.50125258566012,-1.55367636326687,
-0.184119054602967)) ;
#125517=CARTESIAN_POINT('Ctrl Pts',(1.40390259390527,-1.53268199224902,
-0.564273817968124)) ;
#125518=CARTESIAN_POINT('Ctrl Pts',(1.3170642170248,-1.52158568063126,-0.744770163683011)) ;
#125519=CARTESIAN_POINT('Ctrl Pts',(1.08270069078918,-1.50012276598368,
-1.05555862250021)) ;
#125520=CARTESIAN_POINT('Ctrl Pts',(0.939691176779303,-1.48993828925679,
-1.18467241476354)) ;
#125521=CARTESIAN_POINT('Ctrl Pts',(0.606219181844705,-1.47097134753674,
-1.38636274940083)) ;
#125522=CARTESIAN_POINT('Ctrl Pts',(0.417340103520255,-1.46068556267227,
-1.45443413180486)) ;
#125523=CARTESIAN_POINT('Ctrl Pts',(0.147424479608115,-1.4456902502327,
-1.49457125502935)) ;
#125524=CARTESIAN_POINT('Ctrl Pts',(0.0736808700220528,-1.44159338303348,
-1.5)) ;
#125525=CARTESIAN_POINT('Ctrl Pts',(0.,-1.43750000136559,-1.5)) ;
#125526=CARTESIAN_POINT('Origin',(1.38777878078145E-16,-6.28125000068279,
-2.77555756156289E-16)) ;
#125527=CARTESIAN_POINT('',(0.981274813826767,-5.7706329375,0.740569452589779)) ;
#125528=CARTESIAN_POINT('Ctrl Pts',(-1.2293670625,-5.46875000068277,3.46250805804971E-13)) ;
#125529=CARTESIAN_POINT('Ctrl Pts',(-1.2293670625,-5.47663542588566,-0.134325140705998)) ;
#125530=CARTESIAN_POINT('Ctrl Pts',(-1.20735998606848,-5.48522354848241,
-0.26791466575826)) ;
#125531=CARTESIAN_POINT('Ctrl Pts',(-1.11207474840861,-5.5049165150107,
-0.548363706932059)) ;
#125532=CARTESIAN_POINT('Ctrl Pts',(-1.03052046597732,-5.51596717534778,
-0.689522005866121)) ;
#125533=CARTESIAN_POINT('Ctrl Pts',(-0.821238183951841,-5.53706027020258,
-0.928005462370774)) ;
#125534=CARTESIAN_POINT('Ctrl Pts',(-0.697163736115499,-5.54649236723724,
-1.02448119159251)) ;
#125535=CARTESIAN_POINT('Ctrl Pts',(-0.41311506452483,-5.56574676517468,
-1.16930744315786)) ;
#125536=CARTESIAN_POINT('Ctrl Pts',(-0.254549227404192,-5.57649523905455,
-1.21372372448782)) ;
#125537=CARTESIAN_POINT('Ctrl Pts',(0.06714482586041,-5.59830145022596,
-1.23786045820561)) ;
#125538=CARTESIAN_POINT('Ctrl Pts',(0.227099237787686,-5.60914404942507,
-1.21870540434508)) ;
#125539=CARTESIAN_POINT('Ctrl Pts',(0.528144905817568,-5.62955059826449,
-1.12116368850811)) ;
#125540=CARTESIAN_POINT('Ctrl Pts',(0.666691868415718,-5.6383493957678,
-1.04473225017952)) ;
#125541=CARTESIAN_POINT('Ctrl Pts',(0.913115375964076,-5.65876020209116,
-0.83931480906913)) ;
#125542=CARTESIAN_POINT('Ctrl Pts',(1.0167778391346,-5.66985341368972,-0.710195830104623)) ;
#125543=CARTESIAN_POINT('Ctrl Pts',(1.1644893331077,-5.69163252737805,-0.424478399462458)) ;
#125544=CARTESIAN_POINT('Ctrl Pts',(1.2093003899459,-5.70211916585118,-0.271714281660297)) ;
#125545=CARTESIAN_POINT('Ctrl Pts',(1.23789882222414,-5.72101542683666,
0.0336648365788081)) ;
#125546=CARTESIAN_POINT('Ctrl Pts',(1.22473007440643,-5.72966378679881,
0.183234920590739)) ;
#125547=CARTESIAN_POINT('Ctrl Pts',(1.14387771782609,-5.74961362474896,
0.476392493957535)) ;
#125548=CARTESIAN_POINT('Ctrl Pts',(1.07470989404902,-5.76019836853254,
0.616765411484169)) ;
#125549=CARTESIAN_POINT('Ctrl Pts',(0.981274813826767,-5.7706329375,0.740569452589778)) ;
#125550=CARTESIAN_POINT('',(0.753945082394938,-5.77063293749981,-0.971035626067536)) ;
#125551=CARTESIAN_POINT('Origin',(-1.72639680329212E-13,-5.77063293749983,
-4.62130334000221E-14)) ;
#125552=CARTESIAN_POINT('Ctrl Pts',(0.753945082396521,-5.77063293749993,
-0.971035626066305)) ;
#125553=CARTESIAN_POINT('Ctrl Pts',(0.634608850354497,-5.76114897999618,
-1.06369233492909)) ;
#125554=CARTESIAN_POINT('Ctrl Pts',(0.499255840074009,-5.75259233679917,
-1.13354224868022)) ;
#125555=CARTESIAN_POINT('Ctrl Pts',(0.20144221606974,-5.73240487387017,
-1.22325085756158)) ;
#125556=CARTESIAN_POINT('Ctrl Pts',(0.0407802794899434,-5.72151431471711,
-1.23905218162873)) ;
#125557=CARTESIAN_POINT('Ctrl Pts',(-0.28062497204338,-5.69972768013244,
-1.20795774713924)) ;
#125558=CARTESIAN_POINT('Ctrl Pts',(-0.438175539990935,-5.68904802684083,
-1.16014631737484)) ;
#125559=CARTESIAN_POINT('Ctrl Pts',(-0.71912711227131,-5.67000356751088,
-1.00920294138272)) ;
#125560=CARTESIAN_POINT('Ctrl Pts',(-0.841199147635058,-5.66032534014921,
-0.909976073797117)) ;
#125561=CARTESIAN_POINT('Ctrl Pts',(-1.04554886849715,-5.63911215798865,
-0.666599161392545)) ;
#125562=CARTESIAN_POINT('Ctrl Pts',(-1.12411864786825,-5.62803939565067,
-0.523341259854422)) ;
#125563=CARTESIAN_POINT('Ctrl Pts',(-1.21032348273614,-5.60903436230084,
-0.249368318883973)) ;
#125564=CARTESIAN_POINT('Ctrl Pts',(-1.2293670625,-5.60108550690606,-0.124957485518691)) ;
#125565=CARTESIAN_POINT('Ctrl Pts',(-1.2293670625,-5.59375000068276,4.61644611426948E-13)) ;
#125566=CARTESIAN_POINT('Origin',(0.,18.,0.)) ;
#125567=CARTESIAN_POINT('',(-1.53080849893419E-16,17.65,-1.25)) ;
#125568=CARTESIAN_POINT('Origin',(0.,17.65,0.)) ;
#125569=CARTESIAN_POINT('',(-1.95943487863577E-16,18.,-1.6)) ;
#125570=CARTESIAN_POINT('',(-1.95943487863577E-16,18.,-1.6)) ;
#125571=CARTESIAN_POINT('Origin',(0.,18.,0.)) ;
#125572=CARTESIAN_POINT('Origin',(0.,18.,0.)) ;
#125573=CARTESIAN_POINT('',(-1.53080849893419E-16,12.5,-1.25)) ;
#125574=CARTESIAN_POINT('Origin',(0.,12.5,0.)) ;
#125575=CARTESIAN_POINT('',(-1.53080849893419E-16,18.,-1.25)) ;
#125576=CARTESIAN_POINT('Origin',(0.,12.5,0.)) ;
#125577=CARTESIAN_POINT('',(-1.53107198751854E-15,11.7489242262155,0.)) ;
#125578=CARTESIAN_POINT('',(-1.53080849893419E-16,12.5,-1.25)) ;
#125579=CARTESIAN_POINT('Origin',(0.,-0.1,0.)) ;
#125580=CARTESIAN_POINT('',(-1.95943487863577E-16,0.,-1.6)) ;
#125581=CARTESIAN_POINT('Origin',(0.,0.,0.)) ;
#125582=CARTESIAN_POINT('Origin',(-1.95943487863577E-16,-0.1,-1.6)) ;
#125583=CARTESIAN_POINT('Origin',(0.,-6.,0.)) ;
#125584=CARTESIAN_POINT('',(2.17906421430282E-8,-5.7377404754049,-1.26225952459509)) ;
#125585=CARTESIAN_POINT('Ctrl Pts',(2.1866717776764E-8,-5.73774047449605,
-1.26225952550394)) ;
#125586=CARTESIAN_POINT('Ctrl Pts',(-0.0951280656409561,-5.73375893783556,
-1.26624106381238)) ;
#125587=CARTESIAN_POINT('Ctrl Pts',(-0.190610416698374,-5.72980069988564,
-1.2594456998284)) ;
#125588=CARTESIAN_POINT('Ctrl Pts',(-0.450648170228269,-5.71911673850938,
-1.21081193891058)) ;
#125589=CARTESIAN_POINT('Ctrl Pts',(-0.607374360928914,-5.71318902882096,
-1.14689385528148)) ;
#125590=CARTESIAN_POINT('Ctrl Pts',(-0.895203825302845,-5.70041758644624,
-0.958275366297781)) ;
#125591=CARTESIAN_POINT('Ctrl Pts',(-1.02125376648178,-5.69341610589362,
-0.833639491410614)) ;
#125592=CARTESIAN_POINT('Ctrl Pts',(-1.21006754341351,-5.67981112061703,
-0.552467316470427)) ;
#125593=CARTESIAN_POINT('Ctrl Pts',(-1.27501499197834,-5.67333137756034,
-0.401226892638821)) ;
#125594=CARTESIAN_POINT('Ctrl Pts',(-1.35641798423161,-5.65939991142765,
-0.0370296772463542)) ;
#125595=CARTESIAN_POINT('Ctrl Pts',(-1.34606239437347,-5.65347934071539,
0.146692754942947)) ;
#125596=CARTESIAN_POINT('Ctrl Pts',(-1.28962811685841,-5.6415391541019,
0.462693260701388)) ;
#125597=CARTESIAN_POINT('Ctrl Pts',(-1.22414853729526,-5.63459768074411,
0.630545962613037)) ;
#125598=CARTESIAN_POINT('Ctrl Pts',(-1.03122244096974,-5.62082886886645,
0.933420099928659)) ;
#125599=CARTESIAN_POINT('Ctrl Pts',(-0.904931516807769,-5.61413834418237,
1.06504118805754)) ;
#125600=CARTESIAN_POINT('Ctrl Pts',(-0.683806844472658,-5.60503521401725,
1.21910575872353)) ;
#125601=CARTESIAN_POINT('Ctrl Pts',(-0.60562741341424,-5.60212911291405,
1.26296031260107)) ;
#125602=CARTESIAN_POINT('Ctrl Pts',(-0.362982426443556,-5.59284767566245,
1.3710135518573)) ;
#125603=CARTESIAN_POINT('Ctrl Pts',(-0.189062330338105,-5.58628148087862,
1.41216222698045)) ;
#125604=CARTESIAN_POINT('Ctrl Pts',(0.175704914409963,-5.57270889856158,
1.42883650540158)) ;
#125605=CARTESIAN_POINT('Ctrl Pts',(0.363337370015593,-5.5658338966939,
1.40004302390087)) ;
#125606=CARTESIAN_POINT('Ctrl Pts',(0.734812991615101,-5.55239504200623,
1.26436112246092)) ;
#125607=CARTESIAN_POINT('Ctrl Pts',(0.895294849174838,-5.54655524435109,
1.15743901284809)) ;
#125608=CARTESIAN_POINT('Ctrl Pts',(1.15932714106493,-5.5341022447373,0.916548243459604)) ;
#125609=CARTESIAN_POINT('Ctrl Pts',(1.27259612584018,-5.52731204223573,
0.764558468756784)) ;
#125610=CARTESIAN_POINT('Ctrl Pts',(1.39737099473228,-5.51712872405058,
0.506053099003585)) ;
#125611=CARTESIAN_POINT('Ctrl Pts',(1.43135642621274,-5.51366992565339,
0.412585048988348)) ;
#125612=CARTESIAN_POINT('Ctrl Pts',(1.47795810128641,-5.50725550608955,
0.22838679311422)) ;
#125613=CARTESIAN_POINT('Ctrl Pts',(1.49619812498846,-5.50380187501517,
0.124642988468019)) ;
#125614=CARTESIAN_POINT('Ctrl Pts',(1.50000000000133,-5.49999999999866,
-4.37310951340031E-11)) ;
#125615=CARTESIAN_POINT('',(-1.22464679914735E-16,-6.,-0.999999999999998)) ;
#125616=CARTESIAN_POINT('',(-1.22464679914735E-16,-6.,-0.999999999999998)) ;
#125617=CARTESIAN_POINT('Origin',(0.,-6.,0.)) ;
#125618=CARTESIAN_POINT('Ctrl Pts',(0.753945082395014,-5.77063293749988,
-0.971035626067628)) ;
#125619=CARTESIAN_POINT('Ctrl Pts',(0.660062751113685,-5.76575199098791,
-1.05010851979854)) ;
#125620=CARTESIAN_POINT('Ctrl Pts',(0.56562744963666,-5.76186505079845,
-1.10530231965888)) ;
#125621=CARTESIAN_POINT('Ctrl Pts',(0.388796024291164,-5.75421567817824,
-1.18795136393926)) ;
#125622=CARTESIAN_POINT('Ctrl Pts',(0.291380801751046,-5.75004165425893,
-1.21979558247614)) ;
#125623=CARTESIAN_POINT('Ctrl Pts',(0.12800248544407,-5.7431151491797,-1.25200515595124)) ;
#125624=CARTESIAN_POINT('Ctrl Pts',(0.0640816264084869,-5.74042257674819,
-1.25957742214169)) ;
#125625=CARTESIAN_POINT('Ctrl Pts',(2.18667176318559E-8,-5.73774047449605,
-1.26225952550394)) ;
#125626=CARTESIAN_POINT('Ctrl Pts',(0.981274813826771,-5.77063293749999,
0.740569452589782)) ;
#125627=CARTESIAN_POINT('Ctrl Pts',(1.05284908434852,-5.75501478209421,
0.671658180365851)) ;
#125628=CARTESIAN_POINT('Ctrl Pts',(1.11588152236375,-5.7395221143503,0.594367419289388)) ;
#125629=CARTESIAN_POINT('Ctrl Pts',(1.225548935604,-5.70837632247707,0.420996666920777)) ;
#125630=CARTESIAN_POINT('Ctrl Pts',(1.27045943674123,-5.69289700324141,
0.324733598497716)) ;
#125631=CARTESIAN_POINT('Ctrl Pts',(1.36480677937284,-5.64992724118353,
0.0294077284638439)) ;
#125632=CARTESIAN_POINT('Ctrl Pts',(1.36961990956584,-5.62856530733333,
-0.152118142611198)) ;
#125633=CARTESIAN_POINT('Ctrl Pts',(1.34936797478974,-5.59217850615072,
-0.423529198806479)) ;
#125634=CARTESIAN_POINT('Ctrl Pts',(1.3200119253903,-5.57359136443191,-0.557140339533079)) ;
#125635=CARTESIAN_POINT('Ctrl Pts',(1.22318730692142,-5.53625530800328,
-0.815863444886249)) ;
#125636=CARTESIAN_POINT('Ctrl Pts',(1.15514201583412,-5.5177094022426,-0.939251833099467)) ;
#125637=CARTESIAN_POINT('Ctrl Pts',(1.07028821955689,-5.5,-1.05094392194718)) ;
#125638=CARTESIAN_POINT('Origin',(0.,18.,0.)) ;
#125639=CARTESIAN_POINT('',(1.40590516189806,17.7519237886467,2.06490082896921)) ;
#125640=CARTESIAN_POINT('',(1.40590516189806,0.248076211353313,2.06490082896921)) ;
#125641=CARTESIAN_POINT('',(1.40590516189806,18.,2.06490082896921)) ;
#125642=CARTESIAN_POINT('',(1.08530399323385,17.7519237886467,2.25)) ;
#125643=CARTESIAN_POINT('Origin',(0.,17.7519237886467,0.)) ;
#125644=CARTESIAN_POINT('',(1.08530399323385,0.248076211353313,2.25)) ;
#125645=CARTESIAN_POINT('',(1.08530399323385,18.,2.25)) ;
#125646=CARTESIAN_POINT('Origin',(0.,0.248076211353313,0.)) ;
#125647=CARTESIAN_POINT('Origin',(0.,18.,0.)) ;
#125648=CARTESIAN_POINT('',(2.49120915513191,0.248076211353313,0.185099171030792)) ;
#125649=CARTESIAN_POINT('',(2.49120915513191,17.7519237886467,0.185099171030793)) ;
#125650=CARTESIAN_POINT('',(2.49120915513191,18.,0.185099171030792)) ;
#125651=CARTESIAN_POINT('',(2.49120915513191,0.248076211353313,-0.185099171030794)) ;
#125652=CARTESIAN_POINT('Origin',(0.,0.248076211353313,0.)) ;
#125653=CARTESIAN_POINT('',(2.49120915513191,17.7519237886467,-0.185099171030793)) ;
#125654=CARTESIAN_POINT('',(2.49120915513191,18.,-0.185099171030794)) ;
#125655=CARTESIAN_POINT('Origin',(0.,17.7519237886467,0.)) ;
#125656=CARTESIAN_POINT('Origin',(0.,18.,0.)) ;
#125657=CARTESIAN_POINT('',(-1.08530399323399,17.7519237886467,2.25)) ;
#125658=CARTESIAN_POINT('',(-1.08530399323385,0.248076211353313,2.25)) ;
#125659=CARTESIAN_POINT('',(-1.08530399323385,18.,2.25)) ;
#125660=CARTESIAN_POINT('',(-1.40590516189806,17.7519237886467,2.06490082896921)) ;
#125661=CARTESIAN_POINT('Origin',(0.,17.7519237886467,0.)) ;
#125662=CARTESIAN_POINT('',(-1.40590516189806,0.248076211353313,2.06490082896921)) ;
#125663=CARTESIAN_POINT('',(-1.40590516189806,18.,2.06490082896921)) ;
#125664=CARTESIAN_POINT('Origin',(0.,0.248076211353313,0.)) ;
#125665=CARTESIAN_POINT('Origin',(0.,18.,0.)) ;
#125666=CARTESIAN_POINT('',(-2.49120915513191,17.7519237886467,0.185099171030792)) ;
#125667=CARTESIAN_POINT('',(-2.49120915513191,0.248076211353313,0.18509917103079)) ;
#125668=CARTESIAN_POINT('',(-2.49120915513191,18.,0.18509917103079)) ;
#125669=CARTESIAN_POINT('',(-2.49120915513191,17.7519237886467,-0.185099171030793)) ;
#125670=CARTESIAN_POINT('Origin',(0.,17.7519237886467,0.)) ;
#125671=CARTESIAN_POINT('',(-2.49120915513191,0.248076211353313,-0.185099171030793)) ;
#125672=CARTESIAN_POINT('',(-2.49120915513191,18.,-0.185099171030793)) ;
#125673=CARTESIAN_POINT('Origin',(0.,0.248076211353313,0.)) ;
#125674=CARTESIAN_POINT('Origin',(0.,18.,0.)) ;
#125675=CARTESIAN_POINT('',(-1.40590516189806,17.7519237886467,-2.06490082896921)) ;
#125676=CARTESIAN_POINT('',(-1.40590516189806,0.248076211353313,-2.06490082896921)) ;
#125677=CARTESIAN_POINT('',(-1.40590516189806,18.,-2.06490082896921)) ;
#125678=CARTESIAN_POINT('',(-1.08530399323385,17.7519237886467,-2.25)) ;
#125679=CARTESIAN_POINT('Origin',(0.,17.7519237886467,0.)) ;
#125680=CARTESIAN_POINT('',(-1.08530399323385,0.248076211353313,-2.25)) ;
#125681=CARTESIAN_POINT('',(-1.08530399323385,18.,-2.25)) ;
#125682=CARTESIAN_POINT('Origin',(0.,0.248076211353313,0.)) ;
#125683=CARTESIAN_POINT('Origin',(0.,18.,0.)) ;
#125684=CARTESIAN_POINT('',(1.08530399323385,17.7519237886467,-2.25)) ;
#125685=CARTESIAN_POINT('',(1.08530399323385,0.248076211353313,-2.25)) ;
#125686=CARTESIAN_POINT('',(1.08530399323385,18.,-2.25)) ;
#125687=CARTESIAN_POINT('',(1.40590516189806,17.7519237886467,-2.06490082896921)) ;
#125688=CARTESIAN_POINT('Origin',(0.,17.7519237886467,0.)) ;
#125689=CARTESIAN_POINT('',(1.40590516189806,0.248076211353313,-2.06490082896921)) ;
#125690=CARTESIAN_POINT('',(1.40590516189806,18.,-2.06490082896921)) ;
#125691=CARTESIAN_POINT('Origin',(0.,0.248076211353313,0.)) ;
#125692=CARTESIAN_POINT('Origin',(0.,0.248076211353313,0.)) ;
#125693=CARTESIAN_POINT('',(1.94855715851499,-5.70547202639737E-15,1.125)) ;
#125694=CARTESIAN_POINT('Ctrl Pts',(2.49120915513191,0.248076211353315,
0.185099171030797)) ;
#125695=CARTESIAN_POINT('Ctrl Pts',(2.20570698889652,-2.99760216648792E-15,
0.679603428621479)) ;
#125696=CARTESIAN_POINT('Ctrl Pts',(1.94855715851498,-5.10230155997917E-16,
1.12500000000001)) ;
#125697=CARTESIAN_POINT('',(1.94855715851499,-6.07033558534708E-15,-1.125)) ;
#125698=CARTESIAN_POINT('Origin',(0.,0.,0.)) ;
#125699=CARTESIAN_POINT('Ctrl Pts',(1.948557158515,2.89130421732174E-15,
-1.12499999999999)) ;
#125700=CARTESIAN_POINT('Ctrl Pts',(2.20570698889652,5.89805981832114E-15,
-0.67960342862147)) ;
#125701=CARTESIAN_POINT('Ctrl Pts',(2.49120915513191,0.248076211353317,
-0.1850991710308)) ;
#125702=CARTESIAN_POINT('Origin',(0.,0.248076211353313,0.)) ;
#125703=CARTESIAN_POINT('',(-1.18674972404001E-21,-3.4888067610237E-15,
2.25)) ;
#125704=CARTESIAN_POINT('Origin',(0.,0.,0.)) ;
#125705=CARTESIAN_POINT('Ctrl Pts',(1.94855715851498,-5.10230155997917E-16,
1.12500000000001)) ;
#125706=CARTESIAN_POINT('Ctrl Pts',(1.69140732813346,2.25514051876985E-15,
1.57039657137853)) ;
#125707=CARTESIAN_POINT('Ctrl Pts',(1.40590516189807,0.248076211353312,
2.0649008289692)) ;
#125708=CARTESIAN_POINT('Ctrl Pts',(1.08530399323385,0.248076211353317,
2.25)) ;
#125709=CARTESIAN_POINT('Ctrl Pts',(0.514299660763062,3.80251385934116E-15,
2.25)) ;
#125710=CARTESIAN_POINT('Ctrl Pts',(8.16368249596716E-15,2.04092062399181E-15,
2.25)) ;
#125711=CARTESIAN_POINT('Origin',(0.,0.248076211353313,0.)) ;
#125712=CARTESIAN_POINT('',(-1.94855715851499,-6.18872890638757E-15,1.125)) ;
#125713=CARTESIAN_POINT('Origin',(0.,0.,0.)) ;
#125714=CARTESIAN_POINT('Ctrl Pts',(8.16368249596716E-15,2.04092062399181E-15,
2.25)) ;
#125715=CARTESIAN_POINT('Ctrl Pts',(-0.514299660763059,1.38777878078145E-16,
2.25)) ;
#125716=CARTESIAN_POINT('Ctrl Pts',(-1.08530399323386,0.248076211353322,
2.25)) ;
#125717=CARTESIAN_POINT('Ctrl Pts',(-1.40590516189806,0.248076211353319,
2.06490082896921)) ;
#125718=CARTESIAN_POINT('Ctrl Pts',(-1.69140732813346,-1.83186799063151E-15,
1.57039657137853)) ;
#125719=CARTESIAN_POINT('Ctrl Pts',(-1.94855715851499,-5.10230155997935E-16,
1.12499999999999)) ;
#125720=CARTESIAN_POINT('Origin',(0.,0.248076211353313,0.)) ;
#125721=CARTESIAN_POINT('',(-1.94855715851499,-6.09408526551492E-15,-1.125)) ;
#125722=CARTESIAN_POINT('Origin',(0.,0.,0.)) ;
#125723=CARTESIAN_POINT('Ctrl Pts',(-1.94855715851499,-5.10230155997935E-16,
1.12499999999999)) ;
#125724=CARTESIAN_POINT('Ctrl Pts',(-2.20570698889652,6.24500451351651E-16,
0.67960342862147)) ;
#125725=CARTESIAN_POINT('Ctrl Pts',(-2.49120915513191,0.248076211353317,
0.185099171030793)) ;
#125726=CARTESIAN_POINT('Ctrl Pts',(-2.49120915513191,0.248076211353319,
-0.185099171030792)) ;
#125727=CARTESIAN_POINT('Ctrl Pts',(-2.20570698889652,-1.38777878078145E-16,
-0.679603428621472)) ;
#125728=CARTESIAN_POINT('Ctrl Pts',(-1.94855715851499,-6.8030687466392E-16,
-1.125)) ;
#125729=CARTESIAN_POINT('Origin',(0.,0.248076211353313,0.)) ;
#125730=CARTESIAN_POINT('',(-3.75579836458312E-16,-3.69604056788555E-15,
-2.25)) ;
#125731=CARTESIAN_POINT('Origin',(0.,0.,0.)) ;
#125732=CARTESIAN_POINT('Ctrl Pts',(-1.94855715851499,-6.8030687466392E-16,
-1.125)) ;
#125733=CARTESIAN_POINT('Ctrl Pts',(-1.69140732813346,-1.42247325030098E-15,
-1.57039657137852)) ;
#125734=CARTESIAN_POINT('Ctrl Pts',(-1.40590516189807,0.248076211353311,
-2.0649008289692)) ;
#125735=CARTESIAN_POINT('Ctrl Pts',(-1.08530399323385,0.248076211353314,
-2.25)) ;
#125736=CARTESIAN_POINT('Ctrl Pts',(-0.514299660763063,-1.08246744900953E-15,
-2.25)) ;
#125737=CARTESIAN_POINT('Ctrl Pts',(-7.99360577730116E-15,-2.21099734265776E-15,
-2.25)) ;
#125738=CARTESIAN_POINT('Origin',(0.,0.248076211353313,0.)) ;
#125739=CARTESIAN_POINT('Origin',(0.,0.,0.)) ;
#125740=CARTESIAN_POINT('Ctrl Pts',(-7.99360577730116E-15,-2.21099734265776E-15,
-2.25)) ;
#125741=CARTESIAN_POINT('Ctrl Pts',(0.514299660763054,-3.43475248243408E-15,
-2.25)) ;
#125742=CARTESIAN_POINT('Ctrl Pts',(1.08530399323385,0.248076211353315,
-2.25)) ;
#125743=CARTESIAN_POINT('Ctrl Pts',(1.40590516189807,0.248076211353319,
-2.06490082896921)) ;
#125744=CARTESIAN_POINT('Ctrl Pts',(1.69140732813347,-4.44089209850067E-16,
-1.57039657137852)) ;
#125745=CARTESIAN_POINT('Ctrl Pts',(1.948557158515,2.89130421732174E-15,
-1.12499999999999)) ;
#125746=CARTESIAN_POINT('Origin',(0.,18.,0.)) ;
#125747=CARTESIAN_POINT('',(1.94855715851499,18.,1.125)) ;
#125748=CARTESIAN_POINT('Ctrl Pts',(1.40590516189807,17.7519237886467,2.0649008289692)) ;
#125749=CARTESIAN_POINT('Ctrl Pts',(1.69140732813345,18.,1.57039657137854)) ;
#125750=CARTESIAN_POINT('Ctrl Pts',(1.94855715851497,18.,1.12500000000003)) ;
#125751=CARTESIAN_POINT('',(0.,18.,2.25)) ;
#125752=CARTESIAN_POINT('Origin',(0.,18.,0.)) ;
#125753=CARTESIAN_POINT('Ctrl Pts',(-2.72122749865572E-14,18.,2.25)) ;
#125754=CARTESIAN_POINT('Ctrl Pts',(0.514299660763043,18.,2.25)) ;
#125755=CARTESIAN_POINT('Ctrl Pts',(1.08530399323385,17.7519237886467,2.25)) ;
#125756=CARTESIAN_POINT('Origin',(0.,18.,0.)) ;
#125757=CARTESIAN_POINT('',(1.94855715851499,18.,-1.125)) ;
#125758=CARTESIAN_POINT('Origin',(0.,18.,0.)) ;
#125759=CARTESIAN_POINT('Ctrl Pts',(1.94855715851497,18.,1.12500000000003)) ;
#125760=CARTESIAN_POINT('Ctrl Pts',(2.20570698889652,18.,0.679603428621478)) ;
#125761=CARTESIAN_POINT('Ctrl Pts',(2.49120915513193,17.7519237886467,0.18509917103077)) ;
#125762=CARTESIAN_POINT('Ctrl Pts',(2.49120915513191,17.7519237886467,-0.185099171030805)) ;
#125763=CARTESIAN_POINT('Ctrl Pts',(2.20570698889653,18.,-0.679603428621451)) ;
#125764=CARTESIAN_POINT('Ctrl Pts',(1.94855715851502,18.,-1.12499999999995)) ;
#125765=CARTESIAN_POINT('Origin',(0.,18.,0.)) ;
#125766=CARTESIAN_POINT('Ctrl Pts',(-1.08530399323398,17.7519237886466,
2.25)) ;
#125767=CARTESIAN_POINT('Ctrl Pts',(-0.514299660763131,18.,2.25)) ;
#125768=CARTESIAN_POINT('Ctrl Pts',(-2.72122749865572E-14,18.,2.25)) ;
#125769=CARTESIAN_POINT('',(-1.94855715851499,18.,1.125)) ;
#125770=CARTESIAN_POINT('Origin',(0.,18.,0.)) ;
#125771=CARTESIAN_POINT('Ctrl Pts',(-1.94855715851499,18.,1.125)) ;
#125772=CARTESIAN_POINT('Ctrl Pts',(-1.69140732813345,18.,1.57039657137854)) ;
#125773=CARTESIAN_POINT('Ctrl Pts',(-1.40590516189804,17.7519237886467,
2.06490082896925)) ;
#125774=CARTESIAN_POINT('Origin',(0.,18.,0.)) ;
#125775=CARTESIAN_POINT('Ctrl Pts',(-2.4912091551319,17.7519237886467,0.185099171030818)) ;
#125776=CARTESIAN_POINT('Ctrl Pts',(-2.20570698889652,18.,0.67960342862148)) ;
#125777=CARTESIAN_POINT('Ctrl Pts',(-1.94855715851499,18.,1.125)) ;
#125778=CARTESIAN_POINT('',(-1.94855715851499,18.,-1.125)) ;
#125779=CARTESIAN_POINT('Origin',(0.,18.,0.)) ;
#125780=CARTESIAN_POINT('Ctrl Pts',(-1.94855715851499,18.,-1.125)) ;
#125781=CARTESIAN_POINT('Ctrl Pts',(-2.20570698889652,18.,-0.679603428621479)) ;
#125782=CARTESIAN_POINT('Ctrl Pts',(-2.49120915513191,17.7519237886467,
-0.185099171030809)) ;
#125783=CARTESIAN_POINT('Origin',(0.,18.,0.)) ;
#125784=CARTESIAN_POINT('Ctrl Pts',(-1.40590516189808,17.7519237886467,
-2.06490082896919)) ;
#125785=CARTESIAN_POINT('Ctrl Pts',(-1.69140732813347,18.,-1.57039657137852)) ;
#125786=CARTESIAN_POINT('Ctrl Pts',(-1.94855715851499,18.,-1.125)) ;
#125787=CARTESIAN_POINT('',(-3.7557864968429E-16,18.,-2.25)) ;
#125788=CARTESIAN_POINT('Origin',(0.,18.,0.)) ;
#125789=CARTESIAN_POINT('Ctrl Pts',(-3.40153437331965E-14,18.,-2.25)) ;
#125790=CARTESIAN_POINT('Ctrl Pts',(-0.514299660763108,18.,-2.25)) ;
#125791=CARTESIAN_POINT('Ctrl Pts',(-1.08530399323392,17.7519237886466,
-2.25)) ;
#125792=CARTESIAN_POINT('Origin',(0.,18.,0.)) ;
#125793=CARTESIAN_POINT('Ctrl Pts',(1.08530399323384,17.7519237886467,-2.25)) ;
#125794=CARTESIAN_POINT('Ctrl Pts',(0.514299660763037,18.,-2.25)) ;
#125795=CARTESIAN_POINT('Ctrl Pts',(-3.40153437331965E-14,18.,-2.25)) ;
#125796=CARTESIAN_POINT('Origin',(0.,18.,0.)) ;
#125797=CARTESIAN_POINT('Ctrl Pts',(1.94855715851502,18.,-1.12499999999995)) ;
#125798=CARTESIAN_POINT('Ctrl Pts',(1.69140732813348,18.,-1.5703965713785)) ;
#125799=CARTESIAN_POINT('Ctrl Pts',(1.40590516189807,17.7519237886467,-2.0649008289692)) ;
#125800=CARTESIAN_POINT('Origin',(0.,18.,0.)) ;
#125801=CARTESIAN_POINT('Origin',(0.,0.,0.)) ;
#125802=CARTESIAN_POINT('Origin',(0.,-6.,0.)) ;
#125803=CARTESIAN_POINT('Origin',(2.59807621135332,-6.,-4.08638347560999E-16)) ;
#125804=CARTESIAN_POINT('Origin',(1.29903810567666,-6.,-2.25)) ;
#125805=CARTESIAN_POINT('Origin',(-1.29903810567666,-6.,-2.25)) ;
#125806=CARTESIAN_POINT('Origin',(-2.59807621135332,-6.,-4.47194905911973E-16)) ;
#125807=CARTESIAN_POINT('Origin',(-1.29903810567666,-6.,2.25)) ;
#125808=CARTESIAN_POINT('Origin',(1.29903810567666,-6.,2.25)) ;
#125809=CARTESIAN_POINT('Ctrl Pts',(1.2293670625,-6.34375000068279,0.)) ;
#125810=CARTESIAN_POINT('Ctrl Pts',(1.2293670625,-6.30208333401613,-0.709775404467235)) ;
#125811=CARTESIAN_POINT('Ctrl Pts',(0.61468353125,-6.26041666734946,-1.06466310670085)) ;
#125812=CARTESIAN_POINT('Ctrl Pts',(8.69224177194317E-17,-6.21875000068279,
-1.41955080893447)) ;
#125813=CARTESIAN_POINT('Ctrl Pts',(-0.61468353125,-6.17708333401613,-1.06466310670085)) ;
#125814=CARTESIAN_POINT('Ctrl Pts',(-1.2293670625,-6.13541666734946,-0.709775404467235)) ;
#125815=CARTESIAN_POINT('Ctrl Pts',(-1.2293670625,-6.09375000068279,-1.50554043806781E-16)) ;
#125816=CARTESIAN_POINT('Ctrl Pts',(-1.2293670625,-6.05208333401613,0.709775404467234)) ;
#125817=CARTESIAN_POINT('Ctrl Pts',(-0.614683531250001,-6.01041666734946,
1.06466310670085)) ;
#125818=CARTESIAN_POINT('Ctrl Pts',(-2.60767253158295E-16,-5.96875000068279,
1.41955080893447)) ;
#125819=CARTESIAN_POINT('Ctrl Pts',(0.614683531249999,-5.92708333401613,
1.06466310670085)) ;
#125820=CARTESIAN_POINT('Ctrl Pts',(1.2293670625,-5.88541666734946,0.709775404467235)) ;
#125821=CARTESIAN_POINT('Ctrl Pts',(1.2293670625,-5.84375000068279,0.)) ;
#125822=CARTESIAN_POINT('Ctrl Pts',(1.2293670625,-5.80208333401613,-0.709775404467235)) ;
#125823=CARTESIAN_POINT('Ctrl Pts',(0.61468353125,-5.76041666734946,-1.06466310670085)) ;
#125824=CARTESIAN_POINT('Ctrl Pts',(8.69224177194317E-17,-5.71875000068279,
-1.41955080893447)) ;
#125825=CARTESIAN_POINT('Ctrl Pts',(-0.61468353125,-5.67708333401613,-1.06466310670085)) ;
#125826=CARTESIAN_POINT('Ctrl Pts',(-1.2293670625,-5.63541666734946,-0.709775404467235)) ;
#125827=CARTESIAN_POINT('Ctrl Pts',(-1.2293670625,-5.59375000068279,-1.50554043806781E-16)) ;
#125828=CARTESIAN_POINT('Ctrl Pts',(-1.2293670625,-5.55208333401613,0.709775404467234)) ;
#125829=CARTESIAN_POINT('Ctrl Pts',(-0.614683531250001,-5.51041666734946,
1.06466310670085)) ;
#125830=CARTESIAN_POINT('Ctrl Pts',(-2.60767253158295E-16,-5.46875000068279,
1.41955080893447)) ;
#125831=CARTESIAN_POINT('Ctrl Pts',(0.614683531249999,-5.42708333401613,
1.06466310670085)) ;
#125832=CARTESIAN_POINT('Ctrl Pts',(1.2293670625,-5.38541666734946,0.709775404467235)) ;
#125833=CARTESIAN_POINT('Ctrl Pts',(1.2293670625,-5.34375000068279,0.)) ;
#125834=CARTESIAN_POINT('Ctrl Pts',(1.2293670625,-5.30208333401613,-0.709775404467235)) ;
#125835=CARTESIAN_POINT('Ctrl Pts',(0.61468353125,-5.26041666734946,-1.06466310670085)) ;
#125836=CARTESIAN_POINT('Ctrl Pts',(8.69224177194317E-17,-5.21875000068279,
-1.41955080893447)) ;
#125837=CARTESIAN_POINT('Ctrl Pts',(-0.61468353125,-5.17708333401613,-1.06466310670085)) ;
#125838=CARTESIAN_POINT('Ctrl Pts',(-1.2293670625,-5.13541666734946,-0.709775404467235)) ;
#125839=CARTESIAN_POINT('Ctrl Pts',(-1.2293670625,-5.09375000068279,-1.50554043806781E-16)) ;
#125840=CARTESIAN_POINT('Ctrl Pts',(-1.2293670625,-5.05208333401613,0.709775404467234)) ;
#125841=CARTESIAN_POINT('Ctrl Pts',(-0.614683531250001,-5.01041666734946,
1.06466310670085)) ;
#125842=CARTESIAN_POINT('Ctrl Pts',(-2.60767253158295E-16,-4.96875000068279,
1.41955080893447)) ;
#125843=CARTESIAN_POINT('Ctrl Pts',(0.614683531249999,-4.92708333401613,
1.06466310670085)) ;
#125844=CARTESIAN_POINT('Ctrl Pts',(1.2293670625,-4.88541666734946,0.709775404467235)) ;
#125845=CARTESIAN_POINT('Ctrl Pts',(1.2293670625,-4.84375000068279,0.)) ;
#125846=CARTESIAN_POINT('Ctrl Pts',(1.2293670625,-4.80208333401612,-0.709775404467235)) ;
#125847=CARTESIAN_POINT('Ctrl Pts',(0.61468353125,-4.76041666734946,-1.06466310670085)) ;
#125848=CARTESIAN_POINT('Ctrl Pts',(8.69224177194317E-17,-4.71875000068279,
-1.41955080893447)) ;
#125849=CARTESIAN_POINT('Ctrl Pts',(-0.61468353125,-4.67708333401613,-1.06466310670085)) ;
#125850=CARTESIAN_POINT('Ctrl Pts',(-1.2293670625,-4.63541666734946,-0.709775404467235)) ;
#125851=CARTESIAN_POINT('Ctrl Pts',(-1.2293670625,-4.59375000068279,-1.50554043806781E-16)) ;
#125852=CARTESIAN_POINT('Ctrl Pts',(-1.2293670625,-4.55208333401613,0.709775404467234)) ;
#125853=CARTESIAN_POINT('Ctrl Pts',(-0.614683531250001,-4.51041666734946,
1.06466310670085)) ;
#125854=CARTESIAN_POINT('Ctrl Pts',(-2.60767253158295E-16,-4.46875000068279,
1.41955080893447)) ;
#125855=CARTESIAN_POINT('Ctrl Pts',(0.614683531249999,-4.42708333401613,
1.06466310670085)) ;
#125856=CARTESIAN_POINT('Ctrl Pts',(1.2293670625,-4.38541666734946,0.709775404467235)) ;
#125857=CARTESIAN_POINT('Ctrl Pts',(1.2293670625,-4.34375000068279,0.)) ;
#125858=CARTESIAN_POINT('Ctrl Pts',(1.2293670625,-4.30208333401613,-0.709775404467235)) ;
#125859=CARTESIAN_POINT('Ctrl Pts',(0.61468353125,-4.26041666734946,-1.06466310670085)) ;
#125860=CARTESIAN_POINT('Ctrl Pts',(8.69224177194317E-17,-4.21875000068279,
-1.41955080893447)) ;
#125861=CARTESIAN_POINT('Ctrl Pts',(-0.61468353125,-4.17708333401613,-1.06466310670085)) ;
#125862=CARTESIAN_POINT('Ctrl Pts',(-1.2293670625,-4.13541666734946,-0.709775404467235)) ;
#125863=CARTESIAN_POINT('Ctrl Pts',(-1.2293670625,-4.09375000068279,-1.50554043806781E-16)) ;
#125864=CARTESIAN_POINT('Ctrl Pts',(-1.2293670625,-4.05208333401613,0.709775404467234)) ;
#125865=CARTESIAN_POINT('Ctrl Pts',(-0.614683531250001,-4.01041666734946,
1.06466310670085)) ;
#125866=CARTESIAN_POINT('Ctrl Pts',(-2.60767253158295E-16,-3.96875000068279,
1.41955080893447)) ;
#125867=CARTESIAN_POINT('Ctrl Pts',(0.614683531249999,-3.92708333401613,
1.06466310670085)) ;
#125868=CARTESIAN_POINT('Ctrl Pts',(1.2293670625,-3.88541666734946,0.709775404467235)) ;
#125869=CARTESIAN_POINT('Ctrl Pts',(1.2293670625,-3.84375000068279,0.)) ;
#125870=CARTESIAN_POINT('Ctrl Pts',(1.2293670625,-3.80208333401613,-0.709775404467235)) ;
#125871=CARTESIAN_POINT('Ctrl Pts',(0.61468353125,-3.76041666734946,-1.06466310670085)) ;
#125872=CARTESIAN_POINT('Ctrl Pts',(8.69224177194317E-17,-3.71875000068279,
-1.41955080893447)) ;
#125873=CARTESIAN_POINT('Ctrl Pts',(-0.61468353125,-3.67708333401613,-1.06466310670085)) ;
#125874=CARTESIAN_POINT('Ctrl Pts',(-1.2293670625,-3.63541666734946,-0.709775404467235)) ;
#125875=CARTESIAN_POINT('Ctrl Pts',(-1.2293670625,-3.59375000068279,-1.50554043806781E-16)) ;
#125876=CARTESIAN_POINT('Ctrl Pts',(-1.2293670625,-3.55208333401613,0.709775404467234)) ;
#125877=CARTESIAN_POINT('Ctrl Pts',(-0.614683531250001,-3.51041666734946,
1.06466310670085)) ;
#125878=CARTESIAN_POINT('Ctrl Pts',(-2.60767253158295E-16,-3.46875000068279,
1.41955080893447)) ;
#125879=CARTESIAN_POINT('Ctrl Pts',(0.614683531249999,-3.42708333401613,
1.06466310670085)) ;
#125880=CARTESIAN_POINT('Ctrl Pts',(1.2293670625,-3.38541666734946,0.709775404467235)) ;
#125881=CARTESIAN_POINT('Ctrl Pts',(1.2293670625,-3.34375000068279,0.)) ;
#125882=CARTESIAN_POINT('Ctrl Pts',(1.2293670625,-3.30208333401613,-0.709775404467235)) ;
#125883=CARTESIAN_POINT('Ctrl Pts',(0.61468353125,-3.26041666734946,-1.06466310670085)) ;
#125884=CARTESIAN_POINT('Ctrl Pts',(8.69224177194317E-17,-3.21875000068279,
-1.41955080893447)) ;
#125885=CARTESIAN_POINT('Ctrl Pts',(-0.61468353125,-3.17708333401613,-1.06466310670085)) ;
#125886=CARTESIAN_POINT('Ctrl Pts',(-1.2293670625,-3.13541666734946,-0.709775404467235)) ;
#125887=CARTESIAN_POINT('Ctrl Pts',(-1.2293670625,-3.09375000068279,-1.50554043806781E-16)) ;
#125888=CARTESIAN_POINT('Ctrl Pts',(-1.2293670625,-3.05208333401613,0.709775404467234)) ;
#125889=CARTESIAN_POINT('Ctrl Pts',(-0.614683531250001,-3.01041666734946,
1.06466310670085)) ;
#125890=CARTESIAN_POINT('Ctrl Pts',(-2.60767253158295E-16,-2.96875000068279,
1.41955080893447)) ;
#125891=CARTESIAN_POINT('Ctrl Pts',(0.614683531249999,-2.92708333401613,
1.06466310670085)) ;
#125892=CARTESIAN_POINT('Ctrl Pts',(1.2293670625,-2.88541666734946,0.709775404467235)) ;
#125893=CARTESIAN_POINT('Ctrl Pts',(1.2293670625,-2.84375000068279,0.)) ;
#125894=CARTESIAN_POINT('Ctrl Pts',(1.2293670625,-2.80208333401613,-0.709775404467235)) ;
#125895=CARTESIAN_POINT('Ctrl Pts',(0.61468353125,-2.76041666734946,-1.06466310670085)) ;
#125896=CARTESIAN_POINT('Ctrl Pts',(8.69224177194317E-17,-2.71875000068279,
-1.41955080893447)) ;
#125897=CARTESIAN_POINT('Ctrl Pts',(-0.61468353125,-2.67708333401613,-1.06466310670085)) ;
#125898=CARTESIAN_POINT('Ctrl Pts',(-1.2293670625,-2.63541666734946,-0.709775404467235)) ;
#125899=CARTESIAN_POINT('Ctrl Pts',(-1.2293670625,-2.59375000068279,-1.50554043806781E-16)) ;
#125900=CARTESIAN_POINT('Ctrl Pts',(-1.2293670625,-2.55208333401612,0.709775404467234)) ;
#125901=CARTESIAN_POINT('Ctrl Pts',(-0.614683531250001,-2.51041666734946,
1.06466310670085)) ;
#125902=CARTESIAN_POINT('Ctrl Pts',(-2.60767253158295E-16,-2.46875000068279,
1.41955080893447)) ;
#125903=CARTESIAN_POINT('Ctrl Pts',(0.614683531249999,-2.42708333401613,
1.06466310670085)) ;
#125904=CARTESIAN_POINT('Ctrl Pts',(1.2293670625,-2.38541666734946,0.709775404467235)) ;
#125905=CARTESIAN_POINT('Ctrl Pts',(1.2293670625,-2.34375000068279,0.)) ;
#125906=CARTESIAN_POINT('Ctrl Pts',(1.2293670625,-2.30208333401613,-0.709775404467235)) ;
#125907=CARTESIAN_POINT('Ctrl Pts',(0.61468353125,-2.26041666734946,-1.06466310670085)) ;
#125908=CARTESIAN_POINT('Ctrl Pts',(8.69224177194317E-17,-2.21875000068279,
-1.41955080893447)) ;
#125909=CARTESIAN_POINT('Ctrl Pts',(-0.61468353125,-2.17708333401613,-1.06466310670085)) ;
#125910=CARTESIAN_POINT('Ctrl Pts',(-1.2293670625,-2.13541666734946,-0.709775404467235)) ;
#125911=CARTESIAN_POINT('Ctrl Pts',(-1.2293670625,-2.09375000068279,-1.50554043806781E-16)) ;
#125912=CARTESIAN_POINT('Ctrl Pts',(-1.2293670625,-2.05208333401613,0.709775404467234)) ;
#125913=CARTESIAN_POINT('Ctrl Pts',(-0.614683531250001,-2.01041666734946,
1.06466310670085)) ;
#125914=CARTESIAN_POINT('Ctrl Pts',(-2.60767253158295E-16,-1.96875000068279,
1.41955080893447)) ;
#125915=CARTESIAN_POINT('Ctrl Pts',(0.614683531249999,-1.92708333401613,
1.06466310670085)) ;
#125916=CARTESIAN_POINT('Ctrl Pts',(1.2293670625,-1.88541666734946,0.709775404467235)) ;
#125917=CARTESIAN_POINT('Ctrl Pts',(1.2293670625,-1.84375000068279,0.)) ;
#125918=CARTESIAN_POINT('Ctrl Pts',(1.2293670625,-1.80208333401612,-0.709775404467235)) ;
#125919=CARTESIAN_POINT('Ctrl Pts',(0.61468353125,-1.76041666734946,-1.06466310670085)) ;
#125920=CARTESIAN_POINT('Ctrl Pts',(8.69224177194317E-17,-1.71875000068279,
-1.41955080893447)) ;
#125921=CARTESIAN_POINT('Ctrl Pts',(-0.61468353125,-1.67708333401613,-1.06466310670085)) ;
#125922=CARTESIAN_POINT('Ctrl Pts',(-1.2293670625,-1.63541666734946,-0.709775404467235)) ;
#125923=CARTESIAN_POINT('Ctrl Pts',(-1.2293670625,-1.59375000068279,-1.50554043806781E-16)) ;
#125924=CARTESIAN_POINT('Ctrl Pts',(-1.2293670625,-1.55208333401613,0.709775404467234)) ;
#125925=CARTESIAN_POINT('Ctrl Pts',(-0.614683531250001,-1.51041666734946,
1.06466310670085)) ;
#125926=CARTESIAN_POINT('Ctrl Pts',(-2.60767253158295E-16,-1.46875000068279,
1.41955080893447)) ;
#125927=CARTESIAN_POINT('Ctrl Pts',(0.614683531249999,-1.42708333401613,
1.06466310670085)) ;
#125928=CARTESIAN_POINT('Ctrl Pts',(1.2293670625,-1.38541666734946,0.709775404467235)) ;
#125929=CARTESIAN_POINT('Ctrl Pts',(1.2293670625,-1.34375000068279,0.)) ;
#125930=CARTESIAN_POINT('Ctrl Pts',(1.2293670625,-1.30208333401613,-0.709775404467235)) ;
#125931=CARTESIAN_POINT('Ctrl Pts',(0.61468353125,-1.26041666734946,-1.06466310670085)) ;
#125932=CARTESIAN_POINT('Ctrl Pts',(8.69224177194317E-17,-1.21875000068279,
-1.41955080893447)) ;
#125933=CARTESIAN_POINT('Ctrl Pts',(-0.61468353125,-1.17708333401613,-1.06466310670085)) ;
#125934=CARTESIAN_POINT('Ctrl Pts',(-1.2293670625,-1.13541666734946,-0.709775404467235)) ;
#125935=CARTESIAN_POINT('Ctrl Pts',(-1.2293670625,-1.09375000068279,-1.50554043806781E-16)) ;
#125936=CARTESIAN_POINT('Ctrl Pts',(-1.2293670625,-1.05208333401613,0.709775404467234)) ;
#125937=CARTESIAN_POINT('Ctrl Pts',(-0.614683531250001,-1.01041666734946,
1.06466310670085)) ;
#125938=CARTESIAN_POINT('Ctrl Pts',(-2.60767253158295E-16,-0.968750000682792,
1.41955080893447)) ;
#125939=CARTESIAN_POINT('Ctrl Pts',(0.614683531249999,-0.927083334016125,
1.06466310670085)) ;
#125940=CARTESIAN_POINT('Ctrl Pts',(1.2293670625,-0.885416667349459,0.709775404467235)) ;
#125941=CARTESIAN_POINT('Ctrl Pts',(1.2293670625,-0.843750000682792,0.)) ;
#125942=CARTESIAN_POINT('Ctrl Pts',(1.2293670625,-0.832318278700032,-0.1947349222577)) ;
#125943=CARTESIAN_POINT('Ctrl Pts',(1.16918410523995,-0.819406422395166,
-0.37993670843199)) ;
#125944=CARTESIAN_POINT('Ctrl Pts',(1.50001654048127,-6.50000954965131,
0.)) ;
#125945=CARTESIAN_POINT('Ctrl Pts',(1.50001654048127,-6.45834288298464,
-0.866034953435751)) ;
#125946=CARTESIAN_POINT('Ctrl Pts',(0.750008270240635,-6.41667621631797,
-1.29905243015363)) ;
#125947=CARTESIAN_POINT('Ctrl Pts',(1.06058693367482E-16,-6.37500954965132,
-1.73206990687151)) ;
#125948=CARTESIAN_POINT('Ctrl Pts',(-0.750008270240634,-6.33334288298464,
-1.29905243015363)) ;
#125949=CARTESIAN_POINT('Ctrl Pts',(-1.50001654048127,-6.29167621631797,
-0.866034953435752)) ;
#125950=CARTESIAN_POINT('Ctrl Pts',(-1.50001654048127,-6.25000954965131,
-1.83699045496847E-16)) ;
#125951=CARTESIAN_POINT('Ctrl Pts',(-1.50001654048127,-6.20834288298464,
0.866034953435751)) ;
#125952=CARTESIAN_POINT('Ctrl Pts',(-0.750008270240635,-6.16667621631797,
1.29905243015363)) ;
#125953=CARTESIAN_POINT('Ctrl Pts',(-3.18176080102445E-16,-6.1250095496513,
1.73206990687151)) ;
#125954=CARTESIAN_POINT('Ctrl Pts',(0.750008270240633,-6.08334288298464,
1.29905243015363)) ;
#125955=CARTESIAN_POINT('Ctrl Pts',(1.50001654048127,-6.04167621631797,
0.866034953435752)) ;
#125956=CARTESIAN_POINT('Ctrl Pts',(1.50001654048127,-6.00000954965131,
0.)) ;
#125957=CARTESIAN_POINT('Ctrl Pts',(1.50001654048127,-5.95834288298464,
-0.866034953435751)) ;
#125958=CARTESIAN_POINT('Ctrl Pts',(0.750008270240635,-5.91667621631797,
-1.29905243015363)) ;
#125959=CARTESIAN_POINT('Ctrl Pts',(1.06058693367482E-16,-5.87500954965131,
-1.73206990687151)) ;
#125960=CARTESIAN_POINT('Ctrl Pts',(-0.750008270240634,-5.83334288298464,
-1.29905243015363)) ;
#125961=CARTESIAN_POINT('Ctrl Pts',(-1.50001654048127,-5.79167621631797,
-0.866034953435752)) ;
#125962=CARTESIAN_POINT('Ctrl Pts',(-1.50001654048127,-5.75000954965131,
-1.83699045496847E-16)) ;
#125963=CARTESIAN_POINT('Ctrl Pts',(-1.50001654048127,-5.70834288298464,
0.866034953435751)) ;
#125964=CARTESIAN_POINT('Ctrl Pts',(-0.750008270240635,-5.66667621631797,
1.29905243015363)) ;
#125965=CARTESIAN_POINT('Ctrl Pts',(-3.18176080102445E-16,-5.62500954965131,
1.73206990687151)) ;
#125966=CARTESIAN_POINT('Ctrl Pts',(0.750008270240633,-5.58334288298464,
1.29905243015363)) ;
#125967=CARTESIAN_POINT('Ctrl Pts',(1.50001654048127,-5.54167621631797,
0.866034953435752)) ;
#125968=CARTESIAN_POINT('Ctrl Pts',(1.50001654048127,-5.50000954965131,
0.)) ;
#125969=CARTESIAN_POINT('Ctrl Pts',(1.50001654048127,-5.45834288298464,
-0.866034953435751)) ;
#125970=CARTESIAN_POINT('Ctrl Pts',(0.750008270240635,-5.41667621631797,
-1.29905243015363)) ;
#125971=CARTESIAN_POINT('Ctrl Pts',(1.06058693367482E-16,-5.37500954965131,
-1.73206990687151)) ;
#125972=CARTESIAN_POINT('Ctrl Pts',(-0.750008270240634,-5.33334288298464,
-1.29905243015363)) ;
#125973=CARTESIAN_POINT('Ctrl Pts',(-1.50001654048127,-5.29167621631797,
-0.866034953435752)) ;
#125974=CARTESIAN_POINT('Ctrl Pts',(-1.50001654048127,-5.25000954965131,
-1.83699045496847E-16)) ;
#125975=CARTESIAN_POINT('Ctrl Pts',(-1.50001654048127,-5.20834288298464,
0.866034953435751)) ;
#125976=CARTESIAN_POINT('Ctrl Pts',(-0.750008270240635,-5.16667621631797,
1.29905243015363)) ;
#125977=CARTESIAN_POINT('Ctrl Pts',(-3.18176080102445E-16,-5.12500954965131,
1.73206990687151)) ;
#125978=CARTESIAN_POINT('Ctrl Pts',(0.750008270240633,-5.08334288298464,
1.29905243015363)) ;
#125979=CARTESIAN_POINT('Ctrl Pts',(1.50001654048127,-5.04167621631797,
0.866034953435752)) ;
#125980=CARTESIAN_POINT('Ctrl Pts',(1.50001654048127,-5.00000954965131,
0.)) ;
#125981=CARTESIAN_POINT('Ctrl Pts',(1.50001654048127,-4.95834288298464,
-0.866034953435751)) ;
#125982=CARTESIAN_POINT('Ctrl Pts',(0.750008270240635,-4.91667621631797,
-1.29905243015363)) ;
#125983=CARTESIAN_POINT('Ctrl Pts',(1.06058693367482E-16,-4.87500954965131,
-1.73206990687151)) ;
#125984=CARTESIAN_POINT('Ctrl Pts',(-0.750008270240634,-4.83334288298464,
-1.29905243015363)) ;
#125985=CARTESIAN_POINT('Ctrl Pts',(-1.50001654048127,-4.79167621631797,
-0.866034953435752)) ;
#125986=CARTESIAN_POINT('Ctrl Pts',(-1.50001654048127,-4.75000954965131,
-1.83699045496847E-16)) ;
#125987=CARTESIAN_POINT('Ctrl Pts',(-1.50001654048127,-4.70834288298464,
0.866034953435751)) ;
#125988=CARTESIAN_POINT('Ctrl Pts',(-0.750008270240635,-4.66667621631797,
1.29905243015363)) ;
#125989=CARTESIAN_POINT('Ctrl Pts',(-3.18176080102445E-16,-4.62500954965131,
1.73206990687151)) ;
#125990=CARTESIAN_POINT('Ctrl Pts',(0.750008270240633,-4.58334288298464,
1.29905243015363)) ;
#125991=CARTESIAN_POINT('Ctrl Pts',(1.50001654048127,-4.54167621631797,
0.866034953435752)) ;
#125992=CARTESIAN_POINT('Ctrl Pts',(1.50001654048127,-4.50000954965131,
0.)) ;
#125993=CARTESIAN_POINT('Ctrl Pts',(1.50001654048127,-4.45834288298464,
-0.866034953435751)) ;
#125994=CARTESIAN_POINT('Ctrl Pts',(0.750008270240635,-4.41667621631797,
-1.29905243015363)) ;
#125995=CARTESIAN_POINT('Ctrl Pts',(1.06058693367482E-16,-4.37500954965131,
-1.73206990687151)) ;
#125996=CARTESIAN_POINT('Ctrl Pts',(-0.750008270240634,-4.33334288298464,
-1.29905243015363)) ;
#125997=CARTESIAN_POINT('Ctrl Pts',(-1.50001654048127,-4.29167621631797,
-0.866034953435752)) ;
#125998=CARTESIAN_POINT('Ctrl Pts',(-1.50001654048127,-4.2500095496513,
-1.83699045496847E-16)) ;
#125999=CARTESIAN_POINT('Ctrl Pts',(-1.50001654048127,-4.20834288298464,
0.866034953435751)) ;
#126000=CARTESIAN_POINT('Ctrl Pts',(-0.750008270240635,-4.16667621631797,
1.29905243015363)) ;
#126001=CARTESIAN_POINT('Ctrl Pts',(-3.18176080102445E-16,-4.12500954965131,
1.73206990687151)) ;
#126002=CARTESIAN_POINT('Ctrl Pts',(0.750008270240633,-4.08334288298464,
1.29905243015363)) ;
#126003=CARTESIAN_POINT('Ctrl Pts',(1.50001654048127,-4.04167621631797,
0.866034953435752)) ;
#126004=CARTESIAN_POINT('Ctrl Pts',(1.50001654048127,-4.0000095496513,0.)) ;
#126005=CARTESIAN_POINT('Ctrl Pts',(1.50001654048127,-3.95834288298464,
-0.866034953435751)) ;
#126006=CARTESIAN_POINT('Ctrl Pts',(0.750008270240635,-3.91667621631797,
-1.29905243015363)) ;
#126007=CARTESIAN_POINT('Ctrl Pts',(1.06058693367482E-16,-3.87500954965131,
-1.73206990687151)) ;
#126008=CARTESIAN_POINT('Ctrl Pts',(-0.750008270240634,-3.83334288298464,
-1.29905243015363)) ;
#126009=CARTESIAN_POINT('Ctrl Pts',(-1.50001654048127,-3.79167621631797,
-0.866034953435752)) ;
#126010=CARTESIAN_POINT('Ctrl Pts',(-1.50001654048127,-3.7500095496513,
-1.83699045496847E-16)) ;
#126011=CARTESIAN_POINT('Ctrl Pts',(-1.50001654048127,-3.70834288298464,
0.866034953435751)) ;
#126012=CARTESIAN_POINT('Ctrl Pts',(-0.750008270240635,-3.66667621631797,
1.29905243015363)) ;
#126013=CARTESIAN_POINT('Ctrl Pts',(-3.18176080102445E-16,-3.62500954965131,
1.73206990687151)) ;
#126014=CARTESIAN_POINT('Ctrl Pts',(0.750008270240633,-3.58334288298464,
1.29905243015363)) ;
#126015=CARTESIAN_POINT('Ctrl Pts',(1.50001654048127,-3.54167621631797,
0.866034953435752)) ;
#126016=CARTESIAN_POINT('Ctrl Pts',(1.50001654048127,-3.50000954965131,
0.)) ;
#126017=CARTESIAN_POINT('Ctrl Pts',(1.50001654048127,-3.45834288298464,
-0.866034953435751)) ;
#126018=CARTESIAN_POINT('Ctrl Pts',(0.750008270240635,-3.41667621631797,
-1.29905243015363)) ;
#126019=CARTESIAN_POINT('Ctrl Pts',(1.06058693367482E-16,-3.3750095496513,
-1.73206990687151)) ;
#126020=CARTESIAN_POINT('Ctrl Pts',(-0.750008270240634,-3.33334288298464,
-1.29905243015363)) ;
#126021=CARTESIAN_POINT('Ctrl Pts',(-1.50001654048127,-3.29167621631797,
-0.866034953435752)) ;
#126022=CARTESIAN_POINT('Ctrl Pts',(-1.50001654048127,-3.2500095496513,
-1.83699045496847E-16)) ;
#126023=CARTESIAN_POINT('Ctrl Pts',(-1.50001654048127,-3.20834288298464,
0.866034953435751)) ;
#126024=CARTESIAN_POINT('Ctrl Pts',(-0.750008270240635,-3.16667621631797,
1.29905243015363)) ;
#126025=CARTESIAN_POINT('Ctrl Pts',(-3.18176080102445E-16,-3.12500954965131,
1.73206990687151)) ;
#126026=CARTESIAN_POINT('Ctrl Pts',(0.750008270240633,-3.08334288298464,
1.29905243015363)) ;
#126027=CARTESIAN_POINT('Ctrl Pts',(1.50001654048127,-3.04167621631797,
0.866034953435752)) ;
#126028=CARTESIAN_POINT('Ctrl Pts',(1.50001654048127,-3.0000095496513,0.)) ;
#126029=CARTESIAN_POINT('Ctrl Pts',(1.50001654048127,-2.95834288298464,
-0.866034953435751)) ;
#126030=CARTESIAN_POINT('Ctrl Pts',(0.750008270240635,-2.91667621631797,
-1.29905243015363)) ;
#126031=CARTESIAN_POINT('Ctrl Pts',(1.06058693367482E-16,-2.87500954965131,
-1.73206990687151)) ;
#126032=CARTESIAN_POINT('Ctrl Pts',(-0.750008270240634,-2.83334288298464,
-1.29905243015363)) ;
#126033=CARTESIAN_POINT('Ctrl Pts',(-1.50001654048127,-2.79167621631797,
-0.866034953435752)) ;
#126034=CARTESIAN_POINT('Ctrl Pts',(-1.50001654048127,-2.75000954965131,
-1.83699045496847E-16)) ;
#126035=CARTESIAN_POINT('Ctrl Pts',(-1.50001654048127,-2.70834288298464,
0.866034953435751)) ;
#126036=CARTESIAN_POINT('Ctrl Pts',(-0.750008270240635,-2.66667621631797,
1.29905243015363)) ;
#126037=CARTESIAN_POINT('Ctrl Pts',(-3.18176080102445E-16,-2.6250095496513,
1.73206990687151)) ;
#126038=CARTESIAN_POINT('Ctrl Pts',(0.750008270240633,-2.58334288298464,
1.29905243015363)) ;
#126039=CARTESIAN_POINT('Ctrl Pts',(1.50001654048127,-2.54167621631797,
0.866034953435752)) ;
#126040=CARTESIAN_POINT('Ctrl Pts',(1.50001654048127,-2.5000095496513,0.)) ;
#126041=CARTESIAN_POINT('Ctrl Pts',(1.50001654048127,-2.45834288298464,
-0.866034953435751)) ;
#126042=CARTESIAN_POINT('Ctrl Pts',(0.750008270240635,-2.41667621631797,
-1.29905243015363)) ;
#126043=CARTESIAN_POINT('Ctrl Pts',(1.06058693367482E-16,-2.3750095496513,
-1.73206990687151)) ;
#126044=CARTESIAN_POINT('Ctrl Pts',(-0.750008270240634,-2.33334288298464,
-1.29905243015363)) ;
#126045=CARTESIAN_POINT('Ctrl Pts',(-1.50001654048127,-2.29167621631797,
-0.866034953435752)) ;
#126046=CARTESIAN_POINT('Ctrl Pts',(-1.50001654048127,-2.25000954965131,
-1.83699045496847E-16)) ;
#126047=CARTESIAN_POINT('Ctrl Pts',(-1.50001654048127,-2.20834288298464,
0.866034953435751)) ;
#126048=CARTESIAN_POINT('Ctrl Pts',(-0.750008270240635,-2.16667621631797,
1.29905243015363)) ;
#126049=CARTESIAN_POINT('Ctrl Pts',(-3.18176080102445E-16,-2.12500954965131,
1.73206990687151)) ;
#126050=CARTESIAN_POINT('Ctrl Pts',(0.750008270240633,-2.08334288298464,
1.29905243015363)) ;
#126051=CARTESIAN_POINT('Ctrl Pts',(1.50001654048127,-2.04167621631797,
0.866034953435752)) ;
#126052=CARTESIAN_POINT('Ctrl Pts',(1.50001654048127,-2.00000954965131,
0.)) ;
#126053=CARTESIAN_POINT('Ctrl Pts',(1.50001654048127,-1.95834288298464,
-0.866034953435751)) ;
#126054=CARTESIAN_POINT('Ctrl Pts',(0.750008270240635,-1.91667621631797,
-1.29905243015363)) ;
#126055=CARTESIAN_POINT('Ctrl Pts',(1.06058693367482E-16,-1.8750095496513,
-1.73206990687151)) ;
#126056=CARTESIAN_POINT('Ctrl Pts',(-0.750008270240634,-1.83334288298464,
-1.29905243015363)) ;
#126057=CARTESIAN_POINT('Ctrl Pts',(-1.50001654048127,-1.79167621631797,
-0.866034953435752)) ;
#126058=CARTESIAN_POINT('Ctrl Pts',(-1.50001654048127,-1.75000954965131,
-1.83699045496847E-16)) ;
#126059=CARTESIAN_POINT('Ctrl Pts',(-1.50001654048127,-1.70834288298464,
0.866034953435751)) ;
#126060=CARTESIAN_POINT('Ctrl Pts',(-0.750008270240635,-1.66667621631797,
1.29905243015363)) ;
#126061=CARTESIAN_POINT('Ctrl Pts',(-3.18176080102445E-16,-1.6250095496513,
1.73206990687151)) ;
#126062=CARTESIAN_POINT('Ctrl Pts',(0.750008270240633,-1.58334288298464,
1.29905243015363)) ;
#126063=CARTESIAN_POINT('Ctrl Pts',(1.50001654048127,-1.54167621631797,
0.866034953435752)) ;
#126064=CARTESIAN_POINT('Ctrl Pts',(1.50001654048127,-1.5000095496513,0.)) ;
#126065=CARTESIAN_POINT('Ctrl Pts',(1.50001654048127,-1.45834288298464,
-0.866034953435751)) ;
#126066=CARTESIAN_POINT('Ctrl Pts',(0.750008270240635,-1.41667621631797,
-1.29905243015363)) ;
#126067=CARTESIAN_POINT('Ctrl Pts',(1.06058693367482E-16,-1.3750095496513,
-1.73206990687151)) ;
#126068=CARTESIAN_POINT('Ctrl Pts',(-0.750008270240634,-1.33334288298464,
-1.29905243015363)) ;
#126069=CARTESIAN_POINT('Ctrl Pts',(-1.50001654048127,-1.29167621631797,
-0.866034953435752)) ;
#126070=CARTESIAN_POINT('Ctrl Pts',(-1.50001654048127,-1.25000954965131,
-1.83699045496847E-16)) ;
#126071=CARTESIAN_POINT('Ctrl Pts',(-1.50001654048127,-1.20834288298464,
0.866034953435751)) ;
#126072=CARTESIAN_POINT('Ctrl Pts',(-0.750008270240635,-1.16667621631797,
1.29905243015363)) ;
#126073=CARTESIAN_POINT('Ctrl Pts',(-3.18176080102445E-16,-1.12500954965131,
1.73206990687151)) ;
#126074=CARTESIAN_POINT('Ctrl Pts',(0.750008270240633,-1.08334288298464,
1.29905243015363)) ;
#126075=CARTESIAN_POINT('Ctrl Pts',(1.50001654048127,-1.04167621631797,
0.866034953435752)) ;
#126076=CARTESIAN_POINT('Ctrl Pts',(1.50001654048127,-1.00000954965131,
0.)) ;
#126077=CARTESIAN_POINT('Ctrl Pts',(1.50001654048127,-0.988577827668548,
-0.237606499560732)) ;
#126078=CARTESIAN_POINT('Ctrl Pts',(1.42658409373784,-0.975665971363682,
-0.46358110963624)) ;
#126079=CARTESIAN_POINT('',(1.42658067231545,-0.975658586206325,-0.463538116421941)) ;
#126080=CARTESIAN_POINT('Ctrl Pts',(1.5,-6.06250000136559,0.)) ;
#126081=CARTESIAN_POINT('Ctrl Pts',(1.5,-6.02083333469892,-0.866025403784439)) ;
#126082=CARTESIAN_POINT('Ctrl Pts',(0.75,-5.97916666803226,-1.29903810567666)) ;
#126083=CARTESIAN_POINT('Ctrl Pts',(1.06057523872491E-16,-5.93750000136559,
-1.73205080756888)) ;
#126084=CARTESIAN_POINT('Ctrl Pts',(-0.75,-5.89583333469892,-1.29903810567666)) ;
#126085=CARTESIAN_POINT('Ctrl Pts',(-1.5,-5.85416666803226,-0.866025403784439)) ;
#126086=CARTESIAN_POINT('Ctrl Pts',(-1.5,-5.81250000136559,-1.83697019872103E-16)) ;
#126087=CARTESIAN_POINT('Ctrl Pts',(-1.5,-5.77083333469892,0.866025403784438)) ;
#126088=CARTESIAN_POINT('Ctrl Pts',(-0.750000000000001,-5.72916666803226,
1.29903810567666)) ;
#126089=CARTESIAN_POINT('Ctrl Pts',(-3.18172571617472E-16,-5.68750000136559,
1.73205080756888)) ;
#126090=CARTESIAN_POINT('Ctrl Pts',(0.749999999999999,-5.64583333469892,
1.29903810567666)) ;
#126091=CARTESIAN_POINT('Ctrl Pts',(1.5,-5.60416666803226,0.86602540378444)) ;
#126092=CARTESIAN_POINT('Ctrl Pts',(1.5,-5.56250000136559,0.)) ;
#126093=CARTESIAN_POINT('Ctrl Pts',(1.5,-5.52083333469892,-0.866025403784439)) ;
#126094=CARTESIAN_POINT('Ctrl Pts',(0.75,-5.47916666803226,-1.29903810567666)) ;
#126095=CARTESIAN_POINT('Ctrl Pts',(1.06057523872491E-16,-5.43750000136559,
-1.73205080756888)) ;
#126096=CARTESIAN_POINT('Ctrl Pts',(-0.75,-5.39583333469892,-1.29903810567666)) ;
#126097=CARTESIAN_POINT('Ctrl Pts',(-1.5,-5.35416666803226,-0.866025403784439)) ;
#126098=CARTESIAN_POINT('Ctrl Pts',(-1.5,-5.31250000136559,-1.83697019872103E-16)) ;
#126099=CARTESIAN_POINT('Ctrl Pts',(-1.5,-5.27083333469892,0.866025403784438)) ;
#126100=CARTESIAN_POINT('Ctrl Pts',(-0.750000000000001,-5.22916666803225,
1.29903810567666)) ;
#126101=CARTESIAN_POINT('Ctrl Pts',(-3.18172571617472E-16,-5.18750000136559,
1.73205080756888)) ;
#126102=CARTESIAN_POINT('Ctrl Pts',(0.749999999999999,-5.14583333469892,
1.29903810567666)) ;
#126103=CARTESIAN_POINT('Ctrl Pts',(1.5,-5.10416666803225,0.86602540378444)) ;
#126104=CARTESIAN_POINT('Ctrl Pts',(1.5,-5.06250000136559,0.)) ;
#126105=CARTESIAN_POINT('Ctrl Pts',(1.5,-5.02083333469892,-0.866025403784439)) ;
#126106=CARTESIAN_POINT('Ctrl Pts',(0.75,-4.97916666803225,-1.29903810567666)) ;
#126107=CARTESIAN_POINT('Ctrl Pts',(1.06057523872491E-16,-4.93750000136559,
-1.73205080756888)) ;
#126108=CARTESIAN_POINT('Ctrl Pts',(-0.75,-4.89583333469892,-1.29903810567666)) ;
#126109=CARTESIAN_POINT('Ctrl Pts',(-1.5,-4.85416666803226,-0.866025403784439)) ;
#126110=CARTESIAN_POINT('Ctrl Pts',(-1.5,-4.81250000136559,-1.83697019872103E-16)) ;
#126111=CARTESIAN_POINT('Ctrl Pts',(-1.5,-4.77083333469892,0.866025403784438)) ;
#126112=CARTESIAN_POINT('Ctrl Pts',(-0.750000000000001,-4.72916666803226,
1.29903810567666)) ;
#126113=CARTESIAN_POINT('Ctrl Pts',(-3.18172571617472E-16,-4.68750000136559,
1.73205080756888)) ;
#126114=CARTESIAN_POINT('Ctrl Pts',(0.749999999999999,-4.64583333469892,
1.29903810567666)) ;
#126115=CARTESIAN_POINT('Ctrl Pts',(1.5,-4.60416666803225,0.86602540378444)) ;
#126116=CARTESIAN_POINT('Ctrl Pts',(1.5,-4.56250000136559,0.)) ;
#126117=CARTESIAN_POINT('Ctrl Pts',(1.5,-4.52083333469892,-0.866025403784439)) ;
#126118=CARTESIAN_POINT('Ctrl Pts',(0.75,-4.47916666803226,-1.29903810567666)) ;
#126119=CARTESIAN_POINT('Ctrl Pts',(1.06057523872491E-16,-4.43750000136559,
-1.73205080756888)) ;
#126120=CARTESIAN_POINT('Ctrl Pts',(-0.75,-4.39583333469892,-1.29903810567666)) ;
#126121=CARTESIAN_POINT('Ctrl Pts',(-1.5,-4.35416666803225,-0.866025403784439)) ;
#126122=CARTESIAN_POINT('Ctrl Pts',(-1.5,-4.31250000136559,-1.83697019872103E-16)) ;
#126123=CARTESIAN_POINT('Ctrl Pts',(-1.5,-4.27083333469892,0.866025403784438)) ;
#126124=CARTESIAN_POINT('Ctrl Pts',(-0.750000000000001,-4.22916666803225,
1.29903810567666)) ;
#126125=CARTESIAN_POINT('Ctrl Pts',(-3.18172571617472E-16,-4.18750000136559,
1.73205080756888)) ;
#126126=CARTESIAN_POINT('Ctrl Pts',(0.749999999999999,-4.14583333469892,
1.29903810567666)) ;
#126127=CARTESIAN_POINT('Ctrl Pts',(1.5,-4.10416666803226,0.86602540378444)) ;
#126128=CARTESIAN_POINT('Ctrl Pts',(1.5,-4.06250000136559,0.)) ;
#126129=CARTESIAN_POINT('Ctrl Pts',(1.5,-4.02083333469892,-0.866025403784439)) ;
#126130=CARTESIAN_POINT('Ctrl Pts',(0.75,-3.97916666803226,-1.29903810567666)) ;
#126131=CARTESIAN_POINT('Ctrl Pts',(1.06057523872491E-16,-3.93750000136559,
-1.73205080756888)) ;
#126132=CARTESIAN_POINT('Ctrl Pts',(-0.75,-3.89583333469892,-1.29903810567666)) ;
#126133=CARTESIAN_POINT('Ctrl Pts',(-1.5,-3.85416666803226,-0.866025403784439)) ;
#126134=CARTESIAN_POINT('Ctrl Pts',(-1.5,-3.81250000136559,-1.83697019872103E-16)) ;
#126135=CARTESIAN_POINT('Ctrl Pts',(-1.5,-3.77083333469892,0.866025403784438)) ;
#126136=CARTESIAN_POINT('Ctrl Pts',(-0.750000000000001,-3.72916666803226,
1.29903810567666)) ;
#126137=CARTESIAN_POINT('Ctrl Pts',(-3.18172571617472E-16,-3.68750000136559,
1.73205080756888)) ;
#126138=CARTESIAN_POINT('Ctrl Pts',(0.749999999999999,-3.64583333469892,
1.29903810567666)) ;
#126139=CARTESIAN_POINT('Ctrl Pts',(1.5,-3.60416666803226,0.86602540378444)) ;
#126140=CARTESIAN_POINT('Ctrl Pts',(1.5,-3.56250000136559,0.)) ;
#126141=CARTESIAN_POINT('Ctrl Pts',(1.5,-3.52083333469892,-0.866025403784439)) ;
#126142=CARTESIAN_POINT('Ctrl Pts',(0.75,-3.47916666803226,-1.29903810567666)) ;
#126143=CARTESIAN_POINT('Ctrl Pts',(1.06057523872491E-16,-3.43750000136559,
-1.73205080756888)) ;
#126144=CARTESIAN_POINT('Ctrl Pts',(-0.75,-3.39583333469892,-1.29903810567666)) ;
#126145=CARTESIAN_POINT('Ctrl Pts',(-1.5,-3.35416666803225,-0.866025403784439)) ;
#126146=CARTESIAN_POINT('Ctrl Pts',(-1.5,-3.31250000136559,-1.83697019872103E-16)) ;
#126147=CARTESIAN_POINT('Ctrl Pts',(-1.5,-3.27083333469892,0.866025403784438)) ;
#126148=CARTESIAN_POINT('Ctrl Pts',(-0.750000000000001,-3.22916666803226,
1.29903810567666)) ;
#126149=CARTESIAN_POINT('Ctrl Pts',(-3.18172571617472E-16,-3.18750000136559,
1.73205080756888)) ;
#126150=CARTESIAN_POINT('Ctrl Pts',(0.749999999999999,-3.14583333469892,
1.29903810567666)) ;
#126151=CARTESIAN_POINT('Ctrl Pts',(1.5,-3.10416666803226,0.86602540378444)) ;
#126152=CARTESIAN_POINT('Ctrl Pts',(1.5,-3.06250000136559,0.)) ;
#126153=CARTESIAN_POINT('Ctrl Pts',(1.5,-3.02083333469892,-0.866025403784439)) ;
#126154=CARTESIAN_POINT('Ctrl Pts',(0.75,-2.97916666803226,-1.29903810567666)) ;
#126155=CARTESIAN_POINT('Ctrl Pts',(1.06057523872491E-16,-2.93750000136559,
-1.73205080756888)) ;
#126156=CARTESIAN_POINT('Ctrl Pts',(-0.75,-2.89583333469892,-1.29903810567666)) ;
#126157=CARTESIAN_POINT('Ctrl Pts',(-1.5,-2.85416666803226,-0.866025403784439)) ;
#126158=CARTESIAN_POINT('Ctrl Pts',(-1.5,-2.81250000136559,-1.83697019872103E-16)) ;
#126159=CARTESIAN_POINT('Ctrl Pts',(-1.5,-2.77083333469892,0.866025403784438)) ;
#126160=CARTESIAN_POINT('Ctrl Pts',(-0.750000000000001,-2.72916666803226,
1.29903810567666)) ;
#126161=CARTESIAN_POINT('Ctrl Pts',(-3.18172571617472E-16,-2.68750000136559,
1.73205080756888)) ;
#126162=CARTESIAN_POINT('Ctrl Pts',(0.749999999999999,-2.64583333469892,
1.29903810567666)) ;
#126163=CARTESIAN_POINT('Ctrl Pts',(1.5,-2.60416666803226,0.86602540378444)) ;
#126164=CARTESIAN_POINT('Ctrl Pts',(1.5,-2.56250000136559,0.)) ;
#126165=CARTESIAN_POINT('Ctrl Pts',(1.5,-2.52083333469892,-0.866025403784439)) ;
#126166=CARTESIAN_POINT('Ctrl Pts',(0.75,-2.47916666803226,-1.29903810567666)) ;
#126167=CARTESIAN_POINT('Ctrl Pts',(1.06057523872491E-16,-2.43750000136559,
-1.73205080756888)) ;
#126168=CARTESIAN_POINT('Ctrl Pts',(-0.75,-2.39583333469892,-1.29903810567666)) ;
#126169=CARTESIAN_POINT('Ctrl Pts',(-1.5,-2.35416666803226,-0.866025403784439)) ;
#126170=CARTESIAN_POINT('Ctrl Pts',(-1.5,-2.31250000136559,-1.83697019872103E-16)) ;
#126171=CARTESIAN_POINT('Ctrl Pts',(-1.5,-2.27083333469892,0.866025403784438)) ;
#126172=CARTESIAN_POINT('Ctrl Pts',(-0.750000000000001,-2.22916666803226,
1.29903810567666)) ;
#126173=CARTESIAN_POINT('Ctrl Pts',(-3.18172571617472E-16,-2.18750000136559,
1.73205080756888)) ;
#126174=CARTESIAN_POINT('Ctrl Pts',(0.749999999999999,-2.14583333469892,
1.29903810567666)) ;
#126175=CARTESIAN_POINT('Ctrl Pts',(1.5,-2.10416666803226,0.86602540378444)) ;
#126176=CARTESIAN_POINT('Ctrl Pts',(1.5,-2.06250000136559,0.)) ;
#126177=CARTESIAN_POINT('Ctrl Pts',(1.5,-2.02083333469892,-0.866025403784439)) ;
#126178=CARTESIAN_POINT('Ctrl Pts',(0.75,-1.97916666803226,-1.29903810567666)) ;
#126179=CARTESIAN_POINT('Ctrl Pts',(1.06057523872491E-16,-1.93750000136559,
-1.73205080756888)) ;
#126180=CARTESIAN_POINT('Ctrl Pts',(-0.75,-1.89583333469892,-1.29903810567666)) ;
#126181=CARTESIAN_POINT('Ctrl Pts',(-1.5,-1.85416666803226,-0.866025403784439)) ;
#126182=CARTESIAN_POINT('Ctrl Pts',(-1.5,-1.81250000136559,-1.83697019872103E-16)) ;
#126183=CARTESIAN_POINT('Ctrl Pts',(-1.5,-1.77083333469892,0.866025403784438)) ;
#126184=CARTESIAN_POINT('Ctrl Pts',(-0.750000000000001,-1.72916666803226,
1.29903810567666)) ;
#126185=CARTESIAN_POINT('Ctrl Pts',(-3.18172571617472E-16,-1.68750000136559,
1.73205080756888)) ;
#126186=CARTESIAN_POINT('Ctrl Pts',(0.749999999999999,-1.64583333469892,
1.29903810567666)) ;
#126187=CARTESIAN_POINT('Ctrl Pts',(1.5,-1.60416666803226,0.86602540378444)) ;
#126188=CARTESIAN_POINT('Ctrl Pts',(1.5,-1.56250000136559,0.)) ;
#126189=CARTESIAN_POINT('Ctrl Pts',(1.5,-1.52083333469892,-0.866025403784439)) ;
#126190=CARTESIAN_POINT('Ctrl Pts',(0.75,-1.47916666803226,-1.29903810567666)) ;
#126191=CARTESIAN_POINT('Ctrl Pts',(1.06057523872491E-16,-1.43750000136559,
-1.73205080756888)) ;
#126192=CARTESIAN_POINT('Ctrl Pts',(-0.75,-1.39583333469892,-1.29903810567666)) ;
#126193=CARTESIAN_POINT('Ctrl Pts',(-1.5,-1.35416666803225,-0.866025403784439)) ;
#126194=CARTESIAN_POINT('Ctrl Pts',(-1.5,-1.31250000136559,-1.83697019872103E-16)) ;
#126195=CARTESIAN_POINT('Ctrl Pts',(-1.5,-1.27083333469892,0.866025403784438)) ;
#126196=CARTESIAN_POINT('Ctrl Pts',(-0.750000000000001,-1.22916666803226,
1.29903810567666)) ;
#126197=CARTESIAN_POINT('Ctrl Pts',(-3.18172571617472E-16,-1.18750000136559,
1.73205080756888)) ;
#126198=CARTESIAN_POINT('Ctrl Pts',(0.749999999999999,-1.14583333469892,
1.29903810567666)) ;
#126199=CARTESIAN_POINT('Ctrl Pts',(1.5,-1.10416666803226,0.86602540378444)) ;
#126200=CARTESIAN_POINT('Ctrl Pts',(1.5,-1.06250000136559,0.)) ;
#126201=CARTESIAN_POINT('Ctrl Pts',(1.5,-1.02083333469892,-0.866025403784439)) ;
#126202=CARTESIAN_POINT('Ctrl Pts',(0.75,-0.979166668032255,-1.29903810567666)) ;
#126203=CARTESIAN_POINT('Ctrl Pts',(1.06057523872491E-16,-0.937500001365588,
-1.73205080756888)) ;
#126204=CARTESIAN_POINT('Ctrl Pts',(-0.75,-0.895833334698922,-1.29903810567666)) ;
#126205=CARTESIAN_POINT('Ctrl Pts',(-1.5,-0.854166668032255,-0.866025403784439)) ;
#126206=CARTESIAN_POINT('Ctrl Pts',(-1.5,-0.812500001365589,-1.83697019872103E-16)) ;
#126207=CARTESIAN_POINT('Ctrl Pts',(-1.5,-0.770833334698922,0.866025403784438)) ;
#126208=CARTESIAN_POINT('Ctrl Pts',(-0.750000000000001,-0.729166668032255,
1.29903810567666)) ;
#126209=CARTESIAN_POINT('Ctrl Pts',(-3.18172571617472E-16,-0.687500001365589,
1.73205080756888)) ;
#126210=CARTESIAN_POINT('Ctrl Pts',(0.749999999999999,-0.645833334698922,
1.29903810567666)) ;
#126211=CARTESIAN_POINT('Ctrl Pts',(1.5,-0.604166668032255,0.86602540378444)) ;
#126212=CARTESIAN_POINT('Ctrl Pts',(1.5,-0.562500001365589,0.)) ;
#126213=CARTESIAN_POINT('Ctrl Pts',(1.5,-0.551068708039016,-0.237594970054175)) ;
#126214=CARTESIAN_POINT('Ctrl Pts',(1.42657373504468,-0.538157367689847,
-0.463559465959517)) ;
#126215=CARTESIAN_POINT('Ctrl Pts',(1.2293670625,-6.21875000068279,0.)) ;
#126216=CARTESIAN_POINT('Ctrl Pts',(1.2293670625,-6.17708333401612,-0.709775404467235)) ;
#126217=CARTESIAN_POINT('Ctrl Pts',(0.61468353125,-6.13541666734946,-1.06466310670085)) ;
#126218=CARTESIAN_POINT('Ctrl Pts',(8.69224177194317E-17,-6.09375000068279,
-1.41955080893447)) ;
#126219=CARTESIAN_POINT('Ctrl Pts',(-0.61468353125,-6.05208333401613,-1.06466310670085)) ;
#126220=CARTESIAN_POINT('Ctrl Pts',(-1.2293670625,-6.01041666734946,-0.709775404467235)) ;
#126221=CARTESIAN_POINT('Ctrl Pts',(-1.2293670625,-5.96875000068279,-1.50554043806781E-16)) ;
#126222=CARTESIAN_POINT('Ctrl Pts',(-1.2293670625,-5.92708333401613,0.709775404467234)) ;
#126223=CARTESIAN_POINT('Ctrl Pts',(-0.614683531250001,-5.88541666734946,
1.06466310670085)) ;
#126224=CARTESIAN_POINT('Ctrl Pts',(-2.60767253158295E-16,-5.84375000068279,
1.41955080893447)) ;
#126225=CARTESIAN_POINT('Ctrl Pts',(0.614683531249999,-5.80208333401612,
1.06466310670085)) ;
#126226=CARTESIAN_POINT('Ctrl Pts',(1.2293670625,-5.76041666734946,0.709775404467235)) ;
#126227=CARTESIAN_POINT('Ctrl Pts',(1.2293670625,-5.71875000068279,0.)) ;
#126228=CARTESIAN_POINT('Ctrl Pts',(1.2293670625,-5.67708333401613,-0.709775404467235)) ;
#126229=CARTESIAN_POINT('Ctrl Pts',(0.61468353125,-5.63541666734946,-1.06466310670085)) ;
#126230=CARTESIAN_POINT('Ctrl Pts',(8.69224177194317E-17,-5.59375000068279,
-1.41955080893447)) ;
#126231=CARTESIAN_POINT('Ctrl Pts',(-0.61468353125,-5.55208333401612,-1.06466310670085)) ;
#126232=CARTESIAN_POINT('Ctrl Pts',(-1.2293670625,-5.51041666734946,-0.709775404467235)) ;
#126233=CARTESIAN_POINT('Ctrl Pts',(-1.2293670625,-5.46875000068279,-1.50554043806781E-16)) ;
#126234=CARTESIAN_POINT('Ctrl Pts',(-1.2293670625,-5.42708333401612,0.709775404467234)) ;
#126235=CARTESIAN_POINT('Ctrl Pts',(-0.614683531250001,-5.38541666734946,
1.06466310670085)) ;
#126236=CARTESIAN_POINT('Ctrl Pts',(-2.60767253158295E-16,-5.34375000068279,
1.41955080893447)) ;
#126237=CARTESIAN_POINT('Ctrl Pts',(0.614683531249999,-5.30208333401613,
1.06466310670085)) ;
#126238=CARTESIAN_POINT('Ctrl Pts',(1.2293670625,-5.26041666734946,0.709775404467235)) ;
#126239=CARTESIAN_POINT('Ctrl Pts',(1.2293670625,-5.21875000068279,0.)) ;
#126240=CARTESIAN_POINT('Ctrl Pts',(1.2293670625,-5.17708333401613,-0.709775404467235)) ;
#126241=CARTESIAN_POINT('Ctrl Pts',(0.61468353125,-5.13541666734946,-1.06466310670085)) ;
#126242=CARTESIAN_POINT('Ctrl Pts',(8.69224177194317E-17,-5.09375000068279,
-1.41955080893447)) ;
#126243=CARTESIAN_POINT('Ctrl Pts',(-0.61468353125,-5.05208333401613,-1.06466310670085)) ;
#126244=CARTESIAN_POINT('Ctrl Pts',(-1.2293670625,-5.01041666734946,-0.709775404467235)) ;
#126245=CARTESIAN_POINT('Ctrl Pts',(-1.2293670625,-4.96875000068279,-1.50554043806781E-16)) ;
#126246=CARTESIAN_POINT('Ctrl Pts',(-1.2293670625,-4.92708333401613,0.709775404467234)) ;
#126247=CARTESIAN_POINT('Ctrl Pts',(-0.614683531250001,-4.88541666734946,
1.06466310670085)) ;
#126248=CARTESIAN_POINT('Ctrl Pts',(-2.60767253158295E-16,-4.84375000068279,
1.41955080893447)) ;
#126249=CARTESIAN_POINT('Ctrl Pts',(0.614683531249999,-4.80208333401612,
1.06466310670085)) ;
#126250=CARTESIAN_POINT('Ctrl Pts',(1.2293670625,-4.76041666734946,0.709775404467235)) ;
#126251=CARTESIAN_POINT('Ctrl Pts',(1.2293670625,-4.71875000068279,0.)) ;
#126252=CARTESIAN_POINT('Ctrl Pts',(1.2293670625,-4.67708333401612,-0.709775404467235)) ;
#126253=CARTESIAN_POINT('Ctrl Pts',(0.61468353125,-4.63541666734946,-1.06466310670085)) ;
#126254=CARTESIAN_POINT('Ctrl Pts',(8.69224177194317E-17,-4.59375000068279,
-1.41955080893447)) ;
#126255=CARTESIAN_POINT('Ctrl Pts',(-0.61468353125,-4.55208333401613,-1.06466310670085)) ;
#126256=CARTESIAN_POINT('Ctrl Pts',(-1.2293670625,-4.51041666734946,-0.709775404467235)) ;
#126257=CARTESIAN_POINT('Ctrl Pts',(-1.2293670625,-4.46875000068279,-1.50554043806781E-16)) ;
#126258=CARTESIAN_POINT('Ctrl Pts',(-1.2293670625,-4.42708333401613,0.709775404467234)) ;
#126259=CARTESIAN_POINT('Ctrl Pts',(-0.614683531250001,-4.38541666734946,
1.06466310670085)) ;
#126260=CARTESIAN_POINT('Ctrl Pts',(-2.60767253158295E-16,-4.34375000068279,
1.41955080893447)) ;
#126261=CARTESIAN_POINT('Ctrl Pts',(0.614683531249999,-4.30208333401613,
1.06466310670085)) ;
#126262=CARTESIAN_POINT('Ctrl Pts',(1.2293670625,-4.26041666734946,0.709775404467235)) ;
#126263=CARTESIAN_POINT('Ctrl Pts',(1.2293670625,-4.21875000068279,0.)) ;
#126264=CARTESIAN_POINT('Ctrl Pts',(1.2293670625,-4.17708333401613,-0.709775404467235)) ;
#126265=CARTESIAN_POINT('Ctrl Pts',(0.61468353125,-4.13541666734946,-1.06466310670085)) ;
#126266=CARTESIAN_POINT('Ctrl Pts',(8.69224177194317E-17,-4.09375000068279,
-1.41955080893447)) ;
#126267=CARTESIAN_POINT('Ctrl Pts',(-0.61468353125,-4.05208333401613,-1.06466310670085)) ;
#126268=CARTESIAN_POINT('Ctrl Pts',(-1.2293670625,-4.01041666734946,-0.709775404467235)) ;
#126269=CARTESIAN_POINT('Ctrl Pts',(-1.2293670625,-3.96875000068279,-1.50554043806781E-16)) ;
#126270=CARTESIAN_POINT('Ctrl Pts',(-1.2293670625,-3.92708333401613,0.709775404467234)) ;
#126271=CARTESIAN_POINT('Ctrl Pts',(-0.614683531250001,-3.88541666734946,
1.06466310670085)) ;
#126272=CARTESIAN_POINT('Ctrl Pts',(-2.60767253158295E-16,-3.84375000068279,
1.41955080893447)) ;
#126273=CARTESIAN_POINT('Ctrl Pts',(0.614683531249999,-3.80208333401613,
1.06466310670085)) ;
#126274=CARTESIAN_POINT('Ctrl Pts',(1.2293670625,-3.76041666734946,0.709775404467235)) ;
#126275=CARTESIAN_POINT('Ctrl Pts',(1.2293670625,-3.71875000068279,0.)) ;
#126276=CARTESIAN_POINT('Ctrl Pts',(1.2293670625,-3.67708333401613,-0.709775404467235)) ;
#126277=CARTESIAN_POINT('Ctrl Pts',(0.61468353125,-3.63541666734946,-1.06466310670085)) ;
#126278=CARTESIAN_POINT('Ctrl Pts',(8.69224177194317E-17,-3.59375000068279,
-1.41955080893447)) ;
#126279=CARTESIAN_POINT('Ctrl Pts',(-0.61468353125,-3.55208333401613,-1.06466310670085)) ;
#126280=CARTESIAN_POINT('Ctrl Pts',(-1.2293670625,-3.51041666734946,-0.709775404467235)) ;
#126281=CARTESIAN_POINT('Ctrl Pts',(-1.2293670625,-3.46875000068279,-1.50554043806781E-16)) ;
#126282=CARTESIAN_POINT('Ctrl Pts',(-1.2293670625,-3.42708333401613,0.709775404467234)) ;
#126283=CARTESIAN_POINT('Ctrl Pts',(-0.614683531250001,-3.38541666734946,
1.06466310670085)) ;
#126284=CARTESIAN_POINT('Ctrl Pts',(-2.60767253158295E-16,-3.34375000068279,
1.41955080893447)) ;
#126285=CARTESIAN_POINT('Ctrl Pts',(0.614683531249999,-3.30208333401613,
1.06466310670085)) ;
#126286=CARTESIAN_POINT('Ctrl Pts',(1.2293670625,-3.26041666734946,0.709775404467235)) ;
#126287=CARTESIAN_POINT('Ctrl Pts',(1.2293670625,-3.21875000068279,0.)) ;
#126288=CARTESIAN_POINT('Ctrl Pts',(1.2293670625,-3.17708333401613,-0.709775404467235)) ;
#126289=CARTESIAN_POINT('Ctrl Pts',(0.61468353125,-3.13541666734946,-1.06466310670085)) ;
#126290=CARTESIAN_POINT('Ctrl Pts',(8.69224177194317E-17,-3.09375000068279,
-1.41955080893447)) ;
#126291=CARTESIAN_POINT('Ctrl Pts',(-0.61468353125,-3.05208333401613,-1.06466310670085)) ;
#126292=CARTESIAN_POINT('Ctrl Pts',(-1.2293670625,-3.01041666734946,-0.709775404467235)) ;
#126293=CARTESIAN_POINT('Ctrl Pts',(-1.2293670625,-2.96875000068279,-1.50554043806781E-16)) ;
#126294=CARTESIAN_POINT('Ctrl Pts',(-1.2293670625,-2.92708333401613,0.709775404467234)) ;
#126295=CARTESIAN_POINT('Ctrl Pts',(-0.614683531250001,-2.88541666734946,
1.06466310670085)) ;
#126296=CARTESIAN_POINT('Ctrl Pts',(-2.60767253158295E-16,-2.84375000068279,
1.41955080893447)) ;
#126297=CARTESIAN_POINT('Ctrl Pts',(0.614683531249999,-2.80208333401613,
1.06466310670085)) ;
#126298=CARTESIAN_POINT('Ctrl Pts',(1.2293670625,-2.76041666734946,0.709775404467235)) ;
#126299=CARTESIAN_POINT('Ctrl Pts',(1.2293670625,-2.71875000068279,0.)) ;
#126300=CARTESIAN_POINT('Ctrl Pts',(1.2293670625,-2.67708333401613,-0.709775404467235)) ;
#126301=CARTESIAN_POINT('Ctrl Pts',(0.61468353125,-2.63541666734946,-1.06466310670085)) ;
#126302=CARTESIAN_POINT('Ctrl Pts',(8.69224177194317E-17,-2.59375000068279,
-1.41955080893447)) ;
#126303=CARTESIAN_POINT('Ctrl Pts',(-0.61468353125,-2.55208333401613,-1.06466310670085)) ;
#126304=CARTESIAN_POINT('Ctrl Pts',(-1.2293670625,-2.51041666734946,-0.709775404467235)) ;
#126305=CARTESIAN_POINT('Ctrl Pts',(-1.2293670625,-2.46875000068279,-1.50554043806781E-16)) ;
#126306=CARTESIAN_POINT('Ctrl Pts',(-1.2293670625,-2.42708333401613,0.709775404467234)) ;
#126307=CARTESIAN_POINT('Ctrl Pts',(-0.614683531250001,-2.38541666734946,
1.06466310670085)) ;
#126308=CARTESIAN_POINT('Ctrl Pts',(-2.60767253158295E-16,-2.34375000068279,
1.41955080893447)) ;
#126309=CARTESIAN_POINT('Ctrl Pts',(0.614683531249999,-2.30208333401613,
1.06466310670085)) ;
#126310=CARTESIAN_POINT('Ctrl Pts',(1.2293670625,-2.26041666734946,0.709775404467235)) ;
#126311=CARTESIAN_POINT('Ctrl Pts',(1.2293670625,-2.21875000068279,0.)) ;
#126312=CARTESIAN_POINT('Ctrl Pts',(1.2293670625,-2.17708333401613,-0.709775404467235)) ;
#126313=CARTESIAN_POINT('Ctrl Pts',(0.61468353125,-2.13541666734946,-1.06466310670085)) ;
#126314=CARTESIAN_POINT('Ctrl Pts',(8.69224177194317E-17,-2.09375000068279,
-1.41955080893447)) ;
#126315=CARTESIAN_POINT('Ctrl Pts',(-0.61468353125,-2.05208333401613,-1.06466310670085)) ;
#126316=CARTESIAN_POINT('Ctrl Pts',(-1.2293670625,-2.01041666734946,-0.709775404467235)) ;
#126317=CARTESIAN_POINT('Ctrl Pts',(-1.2293670625,-1.96875000068279,-1.50554043806781E-16)) ;
#126318=CARTESIAN_POINT('Ctrl Pts',(-1.2293670625,-1.92708333401613,0.709775404467234)) ;
#126319=CARTESIAN_POINT('Ctrl Pts',(-0.614683531250001,-1.88541666734946,
1.06466310670085)) ;
#126320=CARTESIAN_POINT('Ctrl Pts',(-2.60767253158295E-16,-1.84375000068279,
1.41955080893447)) ;
#126321=CARTESIAN_POINT('Ctrl Pts',(0.614683531249999,-1.80208333401613,
1.06466310670085)) ;
#126322=CARTESIAN_POINT('Ctrl Pts',(1.2293670625,-1.76041666734946,0.709775404467235)) ;
#126323=CARTESIAN_POINT('Ctrl Pts',(1.2293670625,-1.71875000068279,0.)) ;
#126324=CARTESIAN_POINT('Ctrl Pts',(1.2293670625,-1.67708333401613,-0.709775404467235)) ;
#126325=CARTESIAN_POINT('Ctrl Pts',(0.61468353125,-1.63541666734946,-1.06466310670085)) ;
#126326=CARTESIAN_POINT('Ctrl Pts',(8.69224177194317E-17,-1.59375000068279,
-1.41955080893447)) ;
#126327=CARTESIAN_POINT('Ctrl Pts',(-0.61468353125,-1.55208333401613,-1.06466310670085)) ;
#126328=CARTESIAN_POINT('Ctrl Pts',(-1.2293670625,-1.51041666734946,-0.709775404467235)) ;
#126329=CARTESIAN_POINT('Ctrl Pts',(-1.2293670625,-1.46875000068279,-1.50554043806781E-16)) ;
#126330=CARTESIAN_POINT('Ctrl Pts',(-1.2293670625,-1.42708333401613,0.709775404467234)) ;
#126331=CARTESIAN_POINT('Ctrl Pts',(-0.614683531250001,-1.38541666734946,
1.06466310670085)) ;
#126332=CARTESIAN_POINT('Ctrl Pts',(-2.60767253158295E-16,-1.34375000068279,
1.41955080893447)) ;
#126333=CARTESIAN_POINT('Ctrl Pts',(0.614683531249999,-1.30208333401613,
1.06466310670085)) ;
#126334=CARTESIAN_POINT('Ctrl Pts',(1.2293670625,-1.26041666734946,0.709775404467235)) ;
#126335=CARTESIAN_POINT('Ctrl Pts',(1.2293670625,-1.21875000068279,0.)) ;
#126336=CARTESIAN_POINT('Ctrl Pts',(1.2293670625,-1.17708333401613,-0.709775404467235)) ;
#126337=CARTESIAN_POINT('Ctrl Pts',(0.61468353125,-1.13541666734946,-1.06466310670085)) ;
#126338=CARTESIAN_POINT('Ctrl Pts',(8.69224177194317E-17,-1.09375000068279,
-1.41955080893447)) ;
#126339=CARTESIAN_POINT('Ctrl Pts',(-0.61468353125,-1.05208333401613,-1.06466310670085)) ;
#126340=CARTESIAN_POINT('Ctrl Pts',(-1.2293670625,-1.01041666734946,-0.709775404467235)) ;
#126341=CARTESIAN_POINT('Ctrl Pts',(-1.2293670625,-0.968750000682792,-1.50554043806781E-16)) ;
#126342=CARTESIAN_POINT('Ctrl Pts',(-1.2293670625,-0.927083334016125,0.709775404467234)) ;
#126343=CARTESIAN_POINT('Ctrl Pts',(-0.614683531250001,-0.885416667349459,
1.06466310670085)) ;
#126344=CARTESIAN_POINT('Ctrl Pts',(-2.60767253158295E-16,-0.843750000682792,
1.41955080893447)) ;
#126345=CARTESIAN_POINT('Ctrl Pts',(0.614683531249999,-0.802083334016125,
1.06466310670085)) ;
#126346=CARTESIAN_POINT('Ctrl Pts',(1.2293670625,-0.760416667349459,0.709775404467235)) ;
#126347=CARTESIAN_POINT('Ctrl Pts',(1.2293670625,-0.718750000682792,0.)) ;
#126348=CARTESIAN_POINT('Ctrl Pts',(1.2293670625,-0.707318707356219,-0.194727620266851)) ;
#126349=CARTESIAN_POINT('Ctrl Pts',(1.16918850806102,-0.694407367007051,
-0.379923159307147)) ;
#126350=CARTESIAN_POINT('',(1.25324553728064,-0.694450928507311,-0.12117112409355)) ;
#126351=CARTESIAN_POINT('Origin',(0.0710244857294275,1.34904687806339,0.12019472536195)) ;
#126352=CARTESIAN_POINT('Ctrl Pts',(1.48723526368499,-0.552750382528326,
-0.19527229821924)) ;
#126353=CARTESIAN_POINT('Ctrl Pts',(1.46320852678865,-0.567307775622241,
-0.187623192231587)) ;
#126354=CARTESIAN_POINT('Ctrl Pts',(1.43917883085798,-0.581865143924219,
-0.179983325197973)) ;
#126355=CARTESIAN_POINT('Ctrl Pts',(1.41514564580341,-0.596422476608758,
-0.17235438796974)) ;
#126356=CARTESIAN_POINT('Ctrl Pts',(1.39111246013927,-0.610979809662529,
-0.164725450548007)) ;
#126357=CARTESIAN_POINT('Ctrl Pts',(1.36707578381675,-0.62553710951487,
-0.157107434118075)) ;
#126358=CARTESIAN_POINT('Ctrl Pts',(1.34303495730321,-0.640094360830228,
-0.149502452876954)) ;
#126359=CARTESIAN_POINT('Ctrl Pts',(1.31311211923601,-0.658213300025925,
-0.140036779055212)) ;
#126360=CARTESIAN_POINT('Ctrl Pts',(1.28318286116683,-0.676332170829035,
-0.130591232118516)) ;
#126361=CARTESIAN_POINT('Ctrl Pts',(1.25324553728064,-0.694450928507311,
-0.12117112409355)) ;
#126362=CARTESIAN_POINT('Origin',(0.963125678325566,-0.975415808634025,
-1.89018765487928)) ;
#126363=CARTESIAN_POINT('',(0.705741417818,-0.819163651371321,-1.80654836425755)) ;
#126364=CARTESIAN_POINT('Origin',(0.70574766896911,-0.694164125798689,-1.8065291234134)) ;
#126365=CARTESIAN_POINT('',(0.70574766896911,-0.694164125798689,-1.8065291234134)) ;
#126366=CARTESIAN_POINT('Origin',(0.963147555709039,-0.537916056909366,
-1.89012031114991)) ;
#126561=UNCERTAINTY_MEASURE_WITH_UNIT(LENGTH_MEASURE(0.01),#126572,
'DISTANCE_ACCURACY_VALUE',
'Maximum model space distance between geometric entities at asserted c
onnectivities') ;
#126563=UNCERTAINTY_MEASURE_WITH_UNIT(LENGTH_MEASURE(0.01),#126572,
'DISTANCE_ACCURACY_VALUE',
'Maximum model space distance between geometric entities at asserted c
onnectivities') ;
#126569=(
GEOMETRIC_REPRESENTATION_CONTEXT(3)
GLOBAL_UNCERTAINTY_ASSIGNED_CONTEXT((#126561))
GLOBAL_UNIT_ASSIGNED_CONTEXT((#126572,#126574,#126575))
REPRESENTATION_CONTEXT('','3D')
) ;
#126571=(
GEOMETRIC_REPRESENTATION_CONTEXT(3)
GLOBAL_UNCERTAINTY_ASSIGNED_CONTEXT((#126563))
GLOBAL_UNIT_ASSIGNED_CONTEXT((#126572,#126574,#126575))
REPRESENTATION_CONTEXT('','3D')
) ;
#126572=(
LENGTH_UNIT()
NAMED_UNIT(*)
SI_UNIT(.MILLI.,.METRE.)
) ;
#126574=(
NAMED_UNIT(*)
PLANE_ANGLE_UNIT()
SI_UNIT($,.RADIAN.)
) ;
#126575=(
NAMED_UNIT(*)
SI_UNIT($,.STERADIAN.)
SOLID_ANGLE_UNIT()
) ;
#126581=SHAPE_DEFINITION_REPRESENTATION(#126588,#126603) ;
#126588=PRODUCT_DEFINITION_SHAPE('',$,#126611) ;
#126603=SHAPE_REPRESENTATION('',(#76669),#126569) ;
#126605=PRODUCT_DEFINITION_CONTEXT('part definition',#126628,'design') ;
#126611=PRODUCT_DEFINITION('Standoff_M3x18','Standoff_M3x18',#126618,#126605) ;
#126618=PRODUCT_DEFINITION_FORMATION('',$,#126635) ;
#126628=APPLICATION_CONTEXT(
'Core Data for Automotive Mechanical Design Process') ;
#126629=PRODUCT_CONTEXT('part definition',#126628,'mechanical') ;
#126635=PRODUCT('Standoff_M3x18','Standoff_M3x18',$,(#126629)) ;
#126644=PRESENTATION_STYLE_ASSIGNMENT((#126653)) ;
#126653=SURFACE_STYLE_USAGE(.BOTH.,#126662) ;
#126662=SURFACE_SIDE_STYLE('',(#126671)) ;
#126671=SURFACE_STYLE_FILL_AREA(#126680) ;
#126680=FILL_AREA_STYLE('Opaque(165,132,0)',(#126689)) ;
#126689=FILL_AREA_STYLE_COLOUR('Opaque(165,132,0)',#126698) ;
#126698=COLOUR_RGB('Opaque(165,132,0)', 0.31764706, 0.68627451, 0.89019608) ;
ENDSEC;
END-ISO-10303-21;
